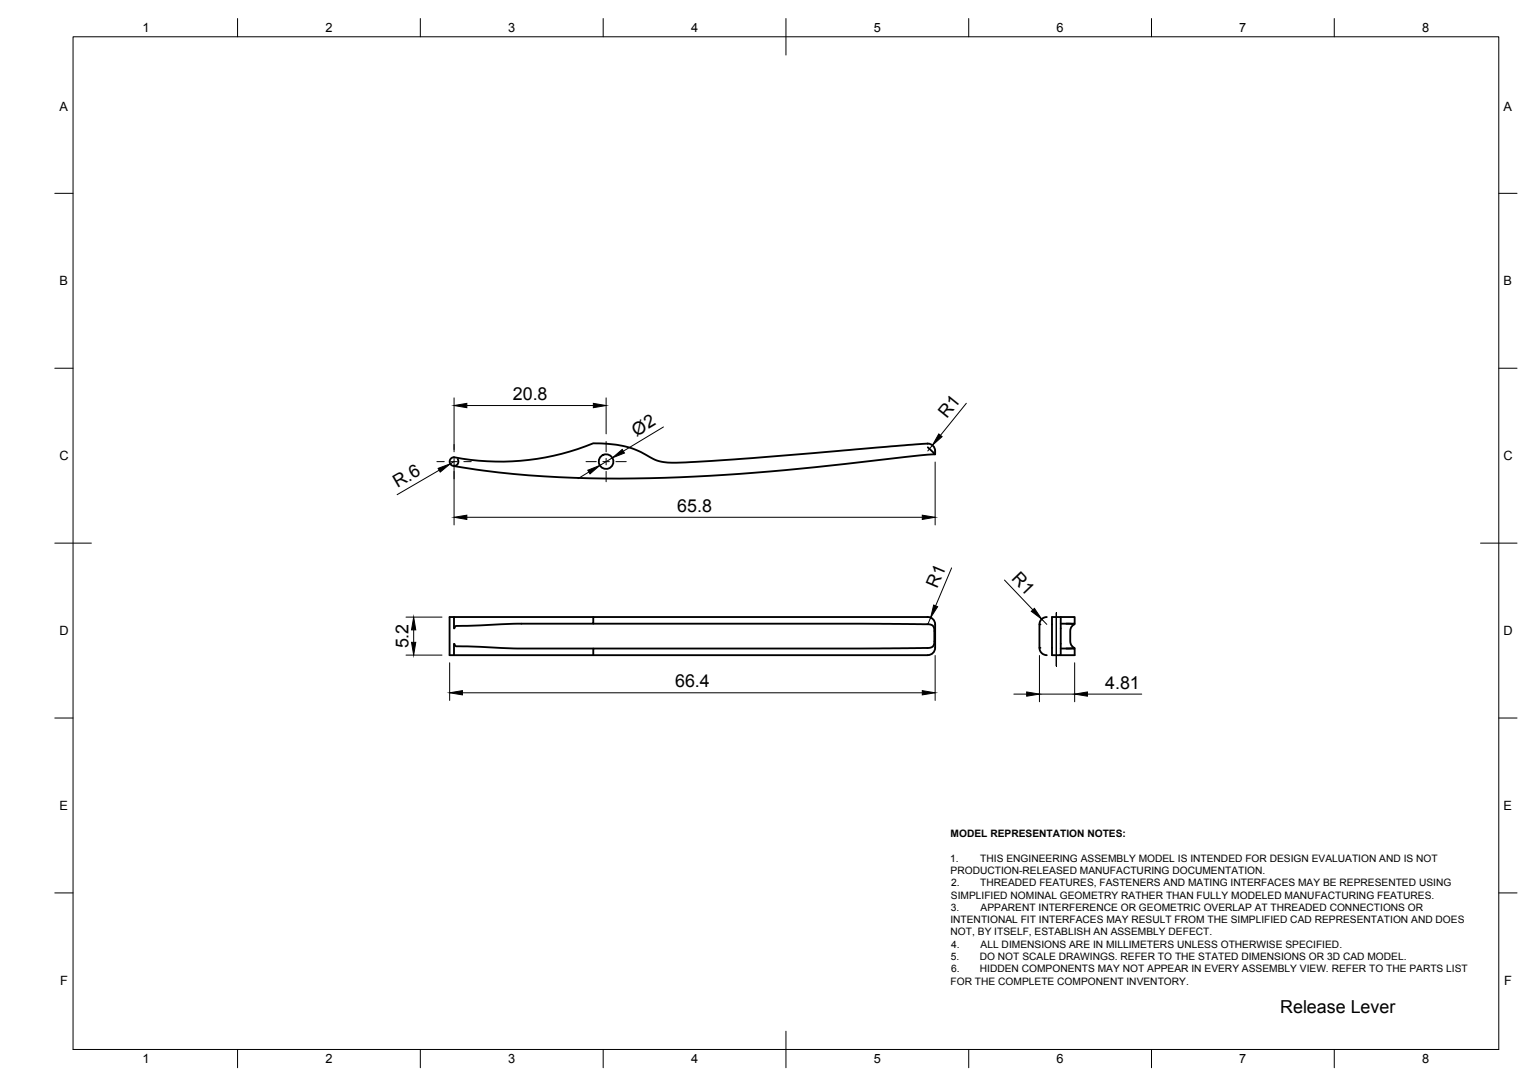
ISO-10303-21;
HEADER;
/* Generated by software containing ST-Developer
 * from STEP Tools, Inc. (www.steptools.com) 
 */

FILE_DESCRIPTION(
/* description */ ('STEP AP214'),
/* implementation_level */ '2;1');

FILE_NAME(
/* name */ 'Release Lever.step',
/* time_stamp */ '2026-10-06T11:11:25-07:00',
/* author */ (''),
/* organization */ (''),
/* preprocessor_version */ 'ST-DEVELOPER v20.2',
/* originating_system */ 'Autodesk Translation Framework v15.15.0.0',
/* authorisation */ '');

FILE_SCHEMA (('AUTOMOTIVE_DESIGN { 1 0 10303 214 3 1 1 }'));
ENDSEC;

DATA;
#10=MECHANICAL_DESIGN_GEOMETRIC_PRESENTATION_REPRESENTATION('',(#708),#47717);
#121=ELLIPSE('',#9861,992.32273705942,143.940737429079);
#122=ELLIPSE('',#9863,1.41421356237156,0.999999999998736);
#123=ELLIPSE('',#9865,1.41421356237466,1.00000000000111);
#133=B_SPLINE_SURFACE_WITH_KNOTS('',3,1,((#46101,#46102),(#46103,#46104),
(#46105,#46106),(#46107,#46108),(#46109,#46110),(#46111,#46112)),
 .UNSPECIFIED.,.F.,.F.,.F.,(4,1,1,4),(2,2),(0.0598879849550618,0.738151675687099,
0.838151675687099,1.),(0.,0.118332698778717),.UNSPECIFIED.);
#134=B_SPLINE_SURFACE_WITH_KNOTS('',3,1,((#46331,#46332),(#46333,#46334),
(#46335,#46336),(#46337,#46338)),.UNSPECIFIED.,.F.,.F.,.F.,(4,4),(2,2),
(0.,0.99999999993505),(0.,0.384000000000005),.UNSPECIFIED.);
#135=B_SPLINE_SURFACE_WITH_KNOTS('',3,1,((#46385,#46386),(#46387,#46388),
(#46389,#46390),(#46391,#46392),(#46393,#46394),(#46395,#46396)),
 .UNSPECIFIED.,.F.,.F.,.F.,(4,1,1,4),(2,2),(0.0598879849550605,0.738151675687099,
0.838151675687099,1.),(0.,0.118332698778627),.UNSPECIFIED.);
#136=B_SPLINE_SURFACE_WITH_KNOTS('',3,1,((#46513,#46514),(#46515,#46516),
(#46517,#46518),(#46519,#46520),(#46521,#46522),(#46523,#46524),(#46525,
#46526),(#46527,#46528),(#46529,#46530),(#46531,#46532),(#46533,#46534),
(#46535,#46536),(#46537,#46538),(#46539,#46540),(#46541,#46542),(#46543,
#46544),(#46545,#46546),(#46547,#46548),(#46549,#46550),(#46551,#46552),
(#46553,#46554),(#46555,#46556)),.UNSPECIFIED.,.F.,.F.,.F.,(4,2,1,1,2,2,
2,2,2,2,2,4),(2,2),(0.,0.00781250000000001,0.015625,0.03125,0.0624999999999999,
0.125,0.25,0.5,0.749999999999999,0.874999999999999,0.9375,1.),(0.,0.412896000000006),
 .UNSPECIFIED.);
#489=B_SPLINE_CURVE_WITH_KNOTS('',3,(#45956,#45957,#45958,#45959,#45960,
#45961),.UNSPECIFIED.,.F.,.F.,(4,2,4),(9.99994026930247E-7,0.0176151554172842,
0.0352487921890912),.UNSPECIFIED.);
#490=B_SPLINE_CURVE_WITH_KNOTS('',3,(#45963,#45964,#45965,#45966,#45967,
#45968,#45969,#45970,#45971,#45972,#45973,#45974,#45975,#45976,#45977,#45978,
#45979,#45980,#45981,#45982,#45983,#45984,#45985,#45986,#45987,#45988,#45989,
#45990,#45991,#45992,#45993,#45994,#45995,#45996,#45997,#45998,#45999,#46000,
#46001,#46002,#46003,#46004,#46005,#46006,#46007,#46008,#46009,#46010,#46011,
#46012,#46013,#46014),.UNSPECIFIED.,.F.,.F.,(4,3,3,3,3,3,3,3,3,3,3,3,3,
3,3,3,3,4),(0.000349648495401886,0.000435856450628066,0.000518346998497937,
0.000600826327770219,0.000683750987549706,0.000694480316306607,0.000804774657733104,
0.000922043397533562,0.00103931213733402,0.00116300366655803,0.00129638856133148,
0.00138414395836143,0.00145781361132506,0.0015307723859531,0.00155655986887515,
0.00162456036766277,0.00169016314809249,0.00172897577938886),
 .UNSPECIFIED.);
#491=B_SPLINE_CURVE_WITH_KNOTS('',3,(#46018,#46019,#46020,#46021,#46022,
#46023,#46024,#46025,#46026,#46027,#46028,#46029,#46030,#46031,#46032,#46033,
#46034,#46035,#46036,#46037,#46038,#46039,#46040,#46041,#46042,#46043,#46044,
#46045,#46046,#46047,#46048,#46049,#46050,#46051,#46052,#46053,#46054,#46055,
#46056,#46057,#46058,#46059,#46060,#46061,#46062,#46063,#46064,#46065,#46066,
#46067,#46068,#46069,#46070,#46071,#46072,#46073,#46074,#46075),
 .UNSPECIFIED.,.F.,.F.,(4,3,3,3,3,3,3,3,3,3,3,3,3,3,3,3,3,3,3,4),(0.,6.18208684431606E-5,
0.000125984546932246,0.00017272653853377,0.000254497619285616,0.000336923412298459,
0.00034545307706754,0.000446850586818363,0.000547260798830634,0.000644898132372486,
0.000690906154135026,0.000804288074237915,0.000913238839396781,0.00101713942033291,
0.00103635923120251,0.00112272247834549,0.00120469306612868,0.0012867711835707,
0.00136943274587814,0.00138181221977441),.UNSPECIFIED.);
#492=B_SPLINE_CURVE_WITH_KNOTS('',3,(#46076,#46077,#46078,#46079,#46080,
#46081),.UNSPECIFIED.,.F.,.F.,(4,2,4),(2.506792132088E-5,0.0175792343156468,
0.0353218856598025),.UNSPECIFIED.);
#493=B_SPLINE_CURVE_WITH_KNOTS('',3,(#46115,#46116,#46117,#46118,#46119,
#46120),.UNSPECIFIED.,.F.,.F.,(4,1,1,4),(0.376076502031257,0.738151675687099,
0.838151675687099,1.),.UNSPECIFIED.);
#494=B_SPLINE_CURVE_WITH_KNOTS('',3,(#46122,#46123,#46124,#46125,#46126,
#46127),.UNSPECIFIED.,.F.,.F.,(4,2,4),(-0.64239307361528,-0.386347437361555,
-6.40648423200219E-10),.UNSPECIFIED.);
#495=B_SPLINE_CURVE_WITH_KNOTS('',3,(#46131,#46132,#46133,#46134,#46135,
#46136),.UNSPECIFIED.,.F.,.F.,(4,1,1,4),(0.0598879851737023,0.738151675687099,
0.838151675687099,1.),.UNSPECIFIED.);
#496=B_SPLINE_CURVE_WITH_KNOTS('',3,(#46142,#46143,#46144,#46145,#46146,
#46147,#46148,#46149,#46150,#46151,#46152,#46153),.UNSPECIFIED.,.F.,.F.,
(4,2,2,2,2,4),(-0.843680482904519,-0.817052168712459,-0.771952825368238,
-0.653804262290151,-0.443525213357367,-1.91323158427181E-7),
 .UNSPECIFIED.);
#497=B_SPLINE_CURVE_WITH_KNOTS('',3,(#46161,#46162,#46163,#46164,#46165,
#46166),.UNSPECIFIED.,.F.,.F.,(4,1,1,4),(0.0598879851737348,0.738151675687099,
0.838151675687099,1.),.UNSPECIFIED.);
#498=B_SPLINE_CURVE_WITH_KNOTS('',3,(#46168,#46169,#46170,#46171,#46172,
#46173,#46174,#46175,#46176,#46177,#46178,#46179,#46180,#46181,#46182,#46183,
#46184,#46185,#46186,#46187,#46188,#46189,#46190,#46191,#46192,#46193,#46194,
#46195,#46196,#46197,#46198,#46199,#46200,#46201,#46202,#46203,#46204,#46205,
#46206,#46207,#46208,#46209,#46210,#46211,#46212,#46213,#46214,#46215,#46216,
#46217,#46218,#46219,#46220,#46221,#46222,#46223,#46224,#46225,#46226,#46227,
#46228,#46229,#46230,#46231,#46232,#46233,#46234,#46235,#46236,#46237,#46238,
#46239,#46240,#46241,#46242,#46243,#46244,#46245,#46246),.UNSPECIFIED.,
 .F.,.F.,(4,3,3,3,3,3,3,3,3,3,3,3,3,3,3,3,3,3,3,3,3,3,3,3,3,3,4),(0.,0.00133019741218274,
0.00338235256079639,0.00652827854954051,0.00749519144790343,0.00804058416816147,
0.0120370484455271,0.0157490242005424,0.0160811683363229,0.0208199774885995,
0.024033074620882,0.0241217525044844,0.0295749122668503,0.0321623366726459,
0.0323411021984972,0.0384974117946658,0.0449050664554913,0.0482435050089688,
0.0490120029708162,0.0550890503579654,0.0562840891771302,0.0573667064243252,
0.060304381261211,0.0615453779150555,0.0623145273032513,0.063632912088931,
0.0643246733452917),.UNSPECIFIED.);
#499=B_SPLINE_CURVE_WITH_KNOTS('',3,(#46252,#46253,#46254,#46255,#46256,
#46257,#46258,#46259,#46260,#46261,#46262,#46263,#46264,#46265,#46266,#46267,
#46268,#46269,#46270,#46271,#46272,#46273,#46274,#46275,#46276,#46277,#46278,
#46279,#46280,#46281,#46282,#46283,#46284,#46285,#46286,#46287,#46288,#46289,
#46290,#46291,#46292,#46293,#46294,#46295,#46296,#46297,#46298,#46299,#46300,
#46301,#46302,#46303,#46304,#46305,#46306,#46307,#46308,#46309,#46310,#46311,
#46312,#46313,#46314,#46315,#46316,#46317,#46318,#46319,#46320,#46321,#46322,
#46323,#46324,#46325,#46326,#46327,#46328,#46329,#46330),.UNSPECIFIED.,
 .F.,.F.,(4,3,3,3,3,3,3,3,3,3,3,3,3,3,3,3,3,3,3,3,3,3,3,3,3,3,4),(0.,0.000694963224053612,
0.00201945044095915,0.00279216000467784,0.0040389008819183,0.0069901733868374,
0.00807780176383661,0.0141829780064518,0.0153835484055692,0.0161556035276732,
0.0226284612866144,0.0288382348705923,0.0321316140743103,0.0323112070553464,
0.0377896082937388,0.040389008819183,0.0404780971676904,0.0452388410930198,
0.0484668105830197,0.0488004921202978,0.0528154549227909,0.0565446123468563,
0.0570925295361479,0.0602530171328019,0.0612244055941231,0.063286059589963,
0.0646224141106929),.UNSPECIFIED.);
#500=B_SPLINE_CURVE_WITH_KNOTS('',3,(#46339,#46340,#46341,#46342,#46343,
#46344,#46345,#46346,#46347,#46348,#46349,#46350,#46351,#46352,#46353,#46354,
#46355,#46356,#46357,#46358,#46359,#46360),.UNSPECIFIED.,.F.,.F.,(4,2,2,
2,2,2,2,2,2,2,4),(0.,0.00822683057377827,0.0164536611475565,0.0246804917213348,
0.0329073222951131,0.0493609834426696,0.0575878140164479,0.061701229303337,
0.0637579369467816,0.0647862907685039,0.0658146445902262),.UNSPECIFIED.);
#501=B_SPLINE_CURVE_WITH_KNOTS('',3,(#46361,#46362,#46363,#46364,#46365,
#46366,#46367,#46368,#46369,#46370,#46371,#46372,#46373,#46374,#46375,#46376,
#46377,#46378,#46379,#46380,#46381,#46382,#46383,#46384),.UNSPECIFIED.,
 .F.,.F.,(4,2,2,2,2,2,2,2,2,2,2,4),(-6.00000000093941E-8,0.00051597907764729,
0.00103201815529459,0.00206409631058923,0.00412825262117847,0.0082565652423569,
0.0165131904847138,0.0330264409694275,0.0412830662117844,0.0495396914541413,
0.0577963166964982,0.0660529419388551),.UNSPECIFIED.);
#502=B_SPLINE_CURVE_WITH_KNOTS('',3,(#46400,#46401,#46402,#46403,#46404,
#46405),.UNSPECIFIED.,.F.,.F.,(4,2,4),(-1.76748570019267,-0.704486820958434,
-1.00000183531384E-6),.UNSPECIFIED.);
#503=B_SPLINE_CURVE_WITH_KNOTS('',3,(#46407,#46408,#46409,#46410,#46411,
#46412),.UNSPECIFIED.,.F.,.F.,(4,1,1,4),(0.376076502030214,0.738151675687099,
0.838151675687099,1.),.UNSPECIFIED.);
#504=B_SPLINE_CURVE_WITH_KNOTS('',3,(#46417,#46418,#46419,#46420,#46421,
#46422,#46423,#46424,#46425,#46426,#46427,#46428),.UNSPECIFIED.,.F.,.F.,
(4,2,2,2,2,4),(-0.957807021571877,-0.464707050841796,-0.230924084318286,
-0.0995694788423429,-0.0494291617315582,-0.0198244706793161),
 .UNSPECIFIED.);
#505=B_SPLINE_CURVE_WITH_KNOTS('',3,(#46430,#46431,#46432,#46433,#46434,
#46435,#46436,#46437,#46438,#46439,#46440,#46441,#46442,#46443,#46444,#46445,
#46446,#46447,#46448,#46449,#46450,#46451,#46452,#46453,#46454,#46455,#46456,
#46457),.UNSPECIFIED.,.F.,.F.,(4,3,3,3,3,3,3,3,3,4),(2.77555756156289E-17,
0.00571779521669806,0.00742042674236585,0.00752642944116232,0.0140544642997195,
0.0148408534847317,0.0186294855440519,0.0236729311553377,0.0285768772393396,
0.0296817069694633),.UNSPECIFIED.);
#506=B_SPLINE_CURVE_WITH_KNOTS('',3,(#46458,#46459,#46460,#46461,#46462,
#46463,#46464,#46465,#46466,#46467,#46468,#46469,#46470),.UNSPECIFIED.,
 .F.,.F.,(4,3,3,3,4),(0.0315167029732621,0.0353810056968997,0.0390981239403465,
0.0415114270041217,0.0422033631272556),.UNSPECIFIED.);
#507=B_SPLINE_CURVE_WITH_KNOTS('',3,(#46472,#46473,#46474,#46475,#46476,
#46477,#46478,#46479,#46480,#46481,#46482,#46483,#46484),.UNSPECIFIED.,
 .F.,.F.,(4,3,3,3,4),(0.,0.000690309032879575,0.00438171613044424,0.00821369103151036,
0.0106615304346148),.UNSPECIFIED.);
#508=B_SPLINE_CURVE_WITH_KNOTS('',3,(#46485,#46486,#46487,#46488,#46489,
#46490,#46491,#46492,#46493,#46494,#46495,#46496,#46497,#46498,#46499,#46500,
#46501,#46502,#46503,#46504,#46505,#46506,#46507,#46508,#46509,#46510,#46511,
#46512),.UNSPECIFIED.,.F.,.F.,(4,3,3,3,3,3,3,3,3,4),(0.0124922114387784,
0.0173786759880834,0.0224014774550337,0.0235184435261858,0.0272981666037043,
0.0338108507614971,0.0345953907531371,0.0347011441861673,0.0404054939590322,
0.0421041217686302),.UNSPECIFIED.);
#509=B_SPLINE_CURVE_WITH_KNOTS('',3,(#46558,#46559,#46560,#46561,#46562,
#46563,#46564,#46565,#46566,#46567,#46568,#46569),.UNSPECIFIED.,.F.,.F.,
(4,2,1,1,2,2,4),(0.,0.00781250000000001,0.015625,0.03125,0.0624999999999999,
0.125,0.242820560992689),.UNSPECIFIED.);
#510=B_SPLINE_CURVE_WITH_KNOTS('',3,(#46571,#46572,#46573,#46574,#46575,
#46576,#46577,#46578,#46579,#46580,#46581,#46582,#46583,#46584,#46585,#46586,
#46587,#46588,#46589,#46590,#46591,#46592,#46593,#46594,#46595,#46596,#46597,
#46598,#46599,#46600,#46601,#46602,#46603,#46604,#46605,#46606,#46607,#46608,
#46609,#46610,#46611,#46612,#46613,#46614,#46615,#46616,#46617,#46618,#46619,
#46620,#46621,#46622,#46623,#46624,#46625,#46626,#46627,#46628),
 .UNSPECIFIED.,.F.,.F.,(4,3,3,3,3,3,3,3,3,3,3,3,3,3,3,3,3,3,3,4),(0.,0.000180857725498468,
0.000242475536420596,0.000462636248961816,0.000484380312649641,0.000484543019812994,
0.000726570468974455,0.000726736566375218,0.000847847927148936,0.000968760625299268,
0.000968976684750301,0.00109011139518026,0.00121095078162408,0.00121122083086588,
0.00145314093794889,0.00145337525175495,0.00167755435588957,0.00169564548526077,
0.00188459038844521,0.00193752125059852),.UNSPECIFIED.);
#511=B_SPLINE_CURVE_WITH_KNOTS('',3,(#46630,#46631,#46632,#46633,#46634,
#46635,#46636,#46637,#46638,#46639,#46640,#46641,#46642,#46643,#46644,#46645,
#46646,#46647),.UNSPECIFIED.,.F.,.F.,(4,2,2,2,2,2,2,2,4),(0.0216871878151901,
0.032680217438002,0.0436732470608138,0.0546662766836257,0.0601627914950316,
0.0629110489007346,0.0642851776035861,0.0649722419550118,0.0656593063064375),
 .UNSPECIFIED.);
#512=B_SPLINE_CURVE_WITH_KNOTS('',3,(#46651,#46652,#46653,#46654,#46655,
#46656,#46657,#46658,#46659,#46660,#46661,#46662,#46663,#46664,#46665,#46666,
#46667,#46668),.UNSPECIFIED.,.F.,.F.,(4,2,2,2,2,2,2,2,4),(0.,0.000689842611306874,
0.00137968522261375,0.00275937044522753,0.00551874089045509,0.0110374817809102,
0.0220749635618205,0.0331124453427309,0.0441499271236412),.UNSPECIFIED.);
#513=B_SPLINE_CURVE_WITH_KNOTS('',3,(#46670,#46671,#46672,#46673,#46674,
#46675,#46676,#46677,#46678,#46679,#46680,#46681,#46682,#46683,#46684,#46685,
#46686,#46687,#46688,#46689,#46690,#46691,#46692,#46693,#46694,#46695,#46696,
#46697,#46698,#46699,#46700,#46701,#46702,#46703,#46704,#46705,#46706,#46707,
#46708,#46709,#46710,#46711,#46712,#46713,#46714,#46715,#46716,#46717,#46718,
#46719,#46720,#46721,#46722,#46723,#46724),.UNSPECIFIED.,.F.,.F.,(4,3,3,
3,3,3,3,3,3,3,3,3,3,3,3,3,3,3,4),(9.33050753687133E-16,0.00018425279266257,
0.000235878931742768,0.000454457410544906,0.000472142579138733,0.000472396351922799,
0.000708293271574268,0.000708594527884195,0.000826400049535313,0.000944531464697737,
0.000944792703845591,0.00106266228766045,0.00118075303404218,0.00118099087980699,
0.0014168040003498,0.00141718905576838,0.00165316656365015,0.001850849561933,
0.00188958540769117),.UNSPECIFIED.);
#514=B_SPLINE_CURVE_WITH_KNOTS('',3,(#46828,#46829,#46830,#46831,#46832,
#46833,#46834,#46835,#46836,#46837,#46838,#46839,#46840,#46841,#46842,#46843,
#46844,#46845,#46846,#46847,#46848,#46849,#46850,#46851,#46852,#46853,#46854,
#46855,#46856,#46857,#46858,#46859,#46860,#46861,#46862,#46863,#46864,#46865,
#46866,#46867,#46868,#46869,#46870,#46871,#46872,#46873,#46874,#46875,#46876),
 .UNSPECIFIED.,.F.,.F.,(4,3,3,3,3,3,3,3,3,3,3,3,3,3,3,3,4),(0.,0.000109468558295443,
0.000219785271344123,0.000330646009385498,0.00044249674566146,0.000468452330512348,
0.000589929933612792,0.000715263674224842,0.000847107675387793,0.000936904661024695,
0.00105512166097558,0.0011758327883036,0.00129946242311971,0.00140535699153704,
0.00158825025111182,0.00178591157987006,0.00187380932204939),
 .UNSPECIFIED.);
#515=B_SPLINE_CURVE_WITH_KNOTS('',3,(#46979,#46980,#46981,#46982,#46983,
#46984,#46985,#46986,#46987,#46988,#46989,#46990,#46991,#46992,#46993,#46994,
#46995,#46996,#46997,#46998,#46999,#47000,#47001,#47002,#47003,#47004,#47005,
#47006,#47007,#47008,#47009,#47010,#47011,#47012,#47013,#47014,#47015,#47016,
#47017,#47018,#47019,#47020,#47021,#47022,#47023,#47024,#47025,#47026,#47027),
 .UNSPECIFIED.,.F.,.F.,(4,3,3,3,3,3,3,3,3,3,3,3,3,3,3,3,4),(-6.33283738354695E-6,
0.000175132894873384,0.000348429481852089,0.000462988112447956,0.00058681834786203,
0.000709001656163456,0.000827259972155947,0.00093230906227946,0.0010641247249674,
0.00119160914162567,0.00131279282513799,0.00140163001211096,0.00151896024956884,
0.0016299235561327,0.00174028554103239,0.00184999846319747,0.00187095096194247),
 .UNSPECIFIED.);
#516=B_SPLINE_CURVE_WITH_KNOTS('',3,(#47033,#47034,#47035,#47036,#47037,
#47038,#47039,#47040,#47041,#47042,#47043,#47044,#47045,#47046,#47047,#47048,
#47049,#47050,#47051,#47052),.UNSPECIFIED.,.F.,.F.,(4,2,2,2,2,2,2,2,2,4),
(1.63264169611634E-6,0.00112071490622925,0.00249410485118844,0.00667587597325017,
0.0315279582548989,0.0586878942058162,0.0843353212386066,0.111794096810849,
0.141395316871198,0.169000061137383),.UNSPECIFIED.);
#517=B_SPLINE_CURVE_WITH_KNOTS('',3,(#47053,#47054,#47055,#47056,#47057,
#47058,#47059,#47060,#47061,#47062,#47063,#47064,#47065,#47066,#47067,#47068,
#47069,#47070,#47071,#47072),.UNSPECIFIED.,.F.,.F.,(4,2,2,2,2,2,2,2,2,4),
(0.,0.0273497535277419,0.0569920982606061,0.0844751673709711,0.110215240941746,
0.137351156959471,0.162388202840594,0.166588867976713,0.167966825157961,
0.169089008366351),.UNSPECIFIED.);
#598=(
BOUNDED_SURFACE()
B_SPLINE_SURFACE(3,2,((#46726,#46727,#46728),(#46729,#46730,#46731),(#46732,
#46733,#46734),(#46735,#46736,#46737),(#46738,#46739,#46740),(#46741,#46742,
#46743),(#46744,#46745,#46746),(#46747,#46748,#46749),(#46750,#46751,#46752),
(#46753,#46754,#46755),(#46756,#46757,#46758),(#46759,#46760,#46761),(#46762,
#46763,#46764),(#46765,#46766,#46767),(#46768,#46769,#46770),(#46771,#46772,
#46773),(#46774,#46775,#46776),(#46777,#46778,#46779),(#46780,#46781,#46782),
(#46783,#46784,#46785),(#46786,#46787,#46788),(#46789,#46790,#46791),(#46792,
#46793,#46794),(#46795,#46796,#46797),(#46798,#46799,#46800),(#46801,#46802,
#46803),(#46804,#46805,#46806),(#46807,#46808,#46809),(#46810,#46811,#46812),
(#46813,#46814,#46815),(#46816,#46817,#46818),(#46819,#46820,#46821),(#46822,
#46823,#46824),(#46825,#46826,#46827)),.UNSPECIFIED.,.F.,.F.,.F.)
B_SPLINE_SURFACE_WITH_KNOTS((4,2,2,2,2,2,2,2,2,2,2,2,2,2,2,2,4),(3,3),(0.0462087893288186,
0.0464703270720222,0.0466010959436241,0.046666480379425,0.0467318648152259,
0.0472549403016333,0.048301091274448,0.0503933932200775,0.0545779971113364,
0.0629472048938543,0.07968562045889,0.0880548282414078,0.0964240360239257,
0.104793243806444,0.108977847697702,0.111070149643332,0.113162451588961),
(0.,1.),.UNSPECIFIED.)
GEOMETRIC_REPRESENTATION_ITEM()
RATIONAL_B_SPLINE_SURFACE(((1.,0.707106781186557,1.),(1.,0.707106781186557,
1.),(1.,0.707106781186551,1.),(1.,0.707106781186551,1.),(1.,0.707106781186557,
1.),(1.,0.707106781186557,1.),(1.,0.707106781186557,1.),(1.,0.707106781186557,
1.),(1.,0.707106781186557,1.),(1.,0.707106781186557,1.),(1.,0.707106781186557,
1.),(1.,0.707106781186557,1.),(1.,0.707106781186557,1.),(1.,0.707106781186557,
1.),(1.,0.707106781186562,1.),(1.,0.707106781186562,1.),(1.,0.707106781186557,
1.),(1.,0.707106781186557,1.),(1.,0.707106781186557,1.),(1.,0.707106781186557,
1.),(1.,0.707106781186557,1.),(1.,0.707106781186557,1.),(1.,0.707106781186538,
1.),(1.,0.707106781186538,1.),(1.,0.707106781186557,1.),(1.,0.707106781186557,
1.),(1.,0.707106781186557,1.),(1.,0.707106781186557,1.),(1.,0.707106781186556,
1.),(1.,0.707106781186556,1.),(1.,0.707106781186557,1.),(1.,0.707106781186557,
1.),(1.,0.707106781186548,1.),(1.,0.707106781186548,1.)))
REPRESENTATION_ITEM('')
SURFACE()
);
#599=(
BOUNDED_SURFACE()
B_SPLINE_SURFACE(3,2,((#46877,#46878,#46879),(#46880,#46881,#46882),(#46883,
#46884,#46885),(#46886,#46887,#46888),(#46889,#46890,#46891),(#46892,#46893,
#46894),(#46895,#46896,#46897),(#46898,#46899,#46900),(#46901,#46902,#46903),
(#46904,#46905,#46906),(#46907,#46908,#46909),(#46910,#46911,#46912),(#46913,
#46914,#46915),(#46916,#46917,#46918),(#46919,#46920,#46921),(#46922,#46923,
#46924),(#46925,#46926,#46927),(#46928,#46929,#46930),(#46931,#46932,#46933),
(#46934,#46935,#46936),(#46937,#46938,#46939),(#46940,#46941,#46942),(#46943,
#46944,#46945),(#46946,#46947,#46948),(#46949,#46950,#46951),(#46952,#46953,
#46954),(#46955,#46956,#46957),(#46958,#46959,#46960),(#46961,#46962,#46963),
(#46964,#46965,#46966),(#46967,#46968,#46969),(#46970,#46971,#46972),(#46973,
#46974,#46975),(#46976,#46977,#46978)),.UNSPECIFIED.,.F.,.F.,.F.)
B_SPLINE_SURFACE_WITH_KNOTS((4,2,2,2,2,2,2,2,2,2,2,2,2,2,2,2,4),(3,3),(0.0317072603307532,
0.0337720562518688,0.0358368521729843,0.0399664440152153,0.0482256276996774,
0.0564848113841394,0.0647439950686015,0.0812623624375256,0.0895215461219877,
0.0936511379642187,0.0957159338853342,0.096748331845892,0.0972645308261708,
0.0973290556987057,0.0973935805712406,0.0975226303163103,0.0977807298064497),
(0.,1.),.UNSPECIFIED.)
GEOMETRIC_REPRESENTATION_ITEM()
RATIONAL_B_SPLINE_SURFACE(((1.,0.707106781186557,1.),(1.,0.707106781186557,
1.),(1.,0.707106781186557,1.),(1.,0.707106781186557,1.),(1.,0.707106781186557,
1.),(1.,0.707106781186557,1.),(1.,0.707106781186556,1.),(1.,0.707106781186556,
1.),(1.,0.707106781186557,1.),(1.,0.707106781186557,1.),(1.,0.707106781186557,
1.),(1.,0.707106781186557,1.),(1.,0.707106781186557,1.),(1.,0.707106781186557,
1.),(1.,0.707106781186557,1.),(1.,0.707106781186557,1.),(1.,0.707106781186553,
1.),(1.,0.707106781186553,1.),(1.,0.707106781186557,1.),(1.,0.707106781186557,
1.),(1.,0.707106781186557,1.),(1.,0.707106781186557,1.),(1.,0.707106781186557,
1.),(1.,0.707106781186557,1.),(1.,0.707106781186557,1.),(1.,0.707106781186557,
1.),(1.,0.707106781186557,1.),(1.,0.707106781186557,1.),(1.,0.707106781186557,
1.),(1.,0.707106781186557,1.),(1.,0.707106781186557,1.),(1.,0.707106781186557,
1.),(1.,0.707106781186557,1.),(1.,0.707106781186557,1.)))
REPRESENTATION_ITEM('')
SURFACE()
);
#600=(
BOUNDED_SURFACE()
B_SPLINE_SURFACE(3,2,((#47073,#47074,#47075),(#47076,#47077,#47078),(#47079,
#47080,#47081),(#47082,#47083,#47084),(#47085,#47086,#47087),(#47088,#47089,
#47090),(#47091,#47092,#47093),(#47094,#47095,#47096),(#47097,#47098,#47099),
(#47100,#47101,#47102),(#47103,#47104,#47105),(#47106,#47107,#47108),(#47109,
#47110,#47111),(#47112,#47113,#47114),(#47115,#47116,#47117),(#47118,#47119,
#47120),(#47121,#47122,#47123),(#47124,#47125,#47126),(#47127,#47128,#47129),
(#47130,#47131,#47132),(#47133,#47134,#47135),(#47136,#47137,#47138)),
 .UNSPECIFIED.,.F.,.F.,.F.)
B_SPLINE_SURFACE_WITH_KNOTS((4,2,2,2,2,2,2,2,2,2,4),(3,3),(0.0497700329860562,
0.0499435417983895,0.0501170506107227,0.0504640682353892,0.0511581034847222,
0.0525461739833882,0.0553223149807202,0.0608745969753841,0.0719791609647121,
0.08308372495404,0.0941882889433679),(0.,1.),.UNSPECIFIED.)
GEOMETRIC_REPRESENTATION_ITEM()
RATIONAL_B_SPLINE_SURFACE(((1.,0.707106781186552,1.),(1.,0.707106781186552,
1.),(1.,0.707106781186548,1.),(1.,0.707106781186548,1.),(1.,0.707106781186548,
1.),(1.,0.707106781186548,1.),(1.,0.707106781186548,1.),(1.,0.707106781186548,
1.),(1.,0.707106781186548,1.),(1.,0.707106781186548,1.),(1.,0.707106781186552,
1.),(1.,0.707106781186552,1.),(1.,0.707106781186552,1.),(1.,0.707106781186552,
1.),(1.,0.707106781186543,1.),(1.,0.707106781186543,1.),(1.,0.707106781186548,
1.),(1.,0.707106781186548,1.),(1.,0.707106781186548,1.),(1.,0.707106781186548,
1.),(1.,0.707106781186548,1.),(1.,0.707106781186548,1.)))
REPRESENTATION_ITEM('')
SURFACE()
);
#601=(
BOUNDED_SURFACE()
B_SPLINE_SURFACE(3,2,((#47140,#47141,#47142),(#47143,#47144,#47145),(#47146,
#47147,#47148),(#47149,#47150,#47151),(#47152,#47153,#47154),(#47155,#47156,
#47157),(#47158,#47159,#47160),(#47161,#47162,#47163),(#47164,#47165,#47166),
(#47167,#47168,#47169),(#47170,#47171,#47172),(#47173,#47174,#47175),(#47176,
#47177,#47178),(#47179,#47180,#47181),(#47182,#47183,#47184),(#47185,#47186,
#47187),(#47188,#47189,#47190),(#47191,#47192,#47193),(#47194,#47195,#47196),
(#47197,#47198,#47199),(#47200,#47201,#47202),(#47203,#47204,#47205)),
 .UNSPECIFIED.,.F.,.F.,.F.)
B_SPLINE_SURFACE_WITH_KNOTS((4,2,2,2,2,2,2,2,2,2,4),(3,3),(0.00146045554386956,
0.00183455394335381,0.0020667680883163,0.00229898223327879,0.00241508930576004,
0.00253119637824129,0.00264730345072254,0.00276341052320378,0.00299562466816628,
0.00322783881312877,0.00360193721261649),(-0.000683445866355827,1.),
 .UNSPECIFIED.)
GEOMETRIC_REPRESENTATION_ITEM()
RATIONAL_B_SPLINE_SURFACE(((1.00042379451114,0.689957513824106,1.),(1.00040554234364,
0.703310559329287,1.),(1.00038207055231,0.720482212916271,1.),(1.00033118410993,
0.75771006437072,1.),(1.00030837452904,0.77439725351972,1.),(1.00025611113095,
0.812632467645312,1.),(1.00022596681978,0.834685648929338,1.),(1.0001846081175,
0.864943131131046,1.),(1.00017167736853,0.874403096882682,1.),(1.00015246067487,
0.88846177701933,1.),(1.00014653964815,0.892793522236095,1.),(1.00014594005926,
0.89323217357368,1.),(1.0001511099939,0.889449917438278,1.),(1.00016917206089,
0.876235946970749,1.),(1.00018188807499,0.866933078428389,1.),(1.0002231052286,
0.836779151366944,1.),(1.00025373494149,0.814370856578693,1.),(1.00030668059841,
0.775636510873654,1.),(1.00032978588761,0.758732985413562,1.),(1.00038153719649,
0.720872409012061,1.),(1.00040541002051,0.7034073651832,1.),(1.00042487779778,
0.689164995581676,1.)))
REPRESENTATION_ITEM('')
SURFACE()
);
#602=(
BOUNDED_SURFACE()
B_SPLINE_SURFACE(3,2,((#47207,#47208,#47209),(#47210,#47211,#47212),(#47213,
#47214,#47215),(#47216,#47217,#47218),(#47219,#47220,#47221),(#47222,#47223,
#47224),(#47225,#47226,#47227),(#47228,#47229,#47230),(#47231,#47232,#47233),
(#47234,#47235,#47236),(#47237,#47238,#47239),(#47240,#47241,#47242)),
 .UNSPECIFIED.,.F.,.F.,.F.)
B_SPLINE_SURFACE_WITH_KNOTS((4,2,2,2,2,4),(3,3),(0.0960380936069649,0.106151670712726,
0.111208459265607,0.113736853542047,0.115001050680268,0.116265247818488),
(0.,1.),.UNSPECIFIED.)
GEOMETRIC_REPRESENTATION_ITEM()
RATIONAL_B_SPLINE_SURFACE(((1.,0.707106781186548,1.),(1.,0.707106781186548,
1.),(1.,0.707106781186548,1.),(1.,0.707106781186548,1.),(1.,0.707106781186557,
1.),(1.,0.707106781186557,1.),(1.,0.707106781186549,1.),(1.,0.707106781186549,
1.),(1.,0.707106781186548,1.),(1.,0.707106781186548,1.),(1.,0.707106781186548,
1.),(1.,0.707106781186548,1.)))
REPRESENTATION_ITEM('')
SURFACE()
);
#603=(
BOUNDED_SURFACE()
B_SPLINE_SURFACE(3,2,((#47243,#47244,#47245),(#47246,#47247,#47248),(#47249,
#47250,#47251),(#47252,#47253,#47254),(#47255,#47256,#47257),(#47258,#47259,
#47260),(#47261,#47262,#47263),(#47264,#47265,#47266),(#47267,#47268,#47269),
(#47270,#47271,#47272),(#47273,#47274,#47275),(#47276,#47277,#47278),(#47279,
#47280,#47281),(#47282,#47283,#47284),(#47285,#47286,#47287),(#47288,#47289,
#47290),(#47291,#47292,#47293),(#47294,#47295,#47296),(#47297,#47298,#47299),
(#47300,#47301,#47302),(#47303,#47304,#47305),(#47306,#47307,#47308)),
 .UNSPECIFIED.,.F.,.F.,.F.)
B_SPLINE_SURFACE_WITH_KNOTS((4,2,2,2,2,2,2,2,2,2,4),(3,3),(0.057360394545972,
0.0683115303997951,0.0792626662536183,0.0902138021074414,0.095689370034353,
0.0984271539978088,0.0997960459795367,0.100480491970401,0.100822714965833,
0.100993826463549,0.101164937961265),(0.,1.),.UNSPECIFIED.)
GEOMETRIC_REPRESENTATION_ITEM()
RATIONAL_B_SPLINE_SURFACE(((1.,0.707106781186537,1.),(1.,0.707106781186537,
1.),(1.,0.707106781186548,1.),(1.,0.707106781186548,1.),(1.,0.707106781186552,
1.),(1.,0.707106781186552,1.),(1.,0.707106781186548,1.),(1.,0.707106781186548,
1.),(1.,0.707106781186548,1.),(1.,0.707106781186548,1.),(1.,0.707106781186549,
1.),(1.,0.707106781186549,1.),(1.,0.707106781186552,1.),(1.,0.707106781186552,
1.),(1.,0.707106781186548,1.),(1.,0.707106781186548,1.),(1.,0.707106781186552,
1.),(1.,0.707106781186552,1.),(1.,0.707106781186548,1.),(1.,0.707106781186548,
1.),(1.,0.707106781186549,1.),(1.,0.707106781186549,1.)))
REPRESENTATION_ITEM('')
SURFACE()
);
#604=(
BOUNDED_SURFACE()
B_SPLINE_SURFACE(3,2,((#47310,#47311,#47312),(#47313,#47314,#47315),(#47316,
#47317,#47318),(#47319,#47320,#47321),(#47322,#47323,#47324),(#47325,#47326,
#47327),(#47328,#47329,#47330),(#47331,#47332,#47333),(#47334,#47335,#47336),
(#47337,#47338,#47339),(#47340,#47341,#47342),(#47343,#47344,#47345),(#47346,
#47347,#47348),(#47349,#47350,#47351),(#47352,#47353,#47354),(#47355,#47356,
#47357),(#47358,#47359,#47360),(#47361,#47362,#47363),(#47364,#47365,#47366),
(#47367,#47368,#47369),(#47370,#47371,#47372),(#47373,#47374,#47375)),
 .UNSPECIFIED.,.F.,.F.,.F.)
B_SPLINE_SURFACE_WITH_KNOTS((4,2,2,2,2,2,2,2,2,2,4),(3,3),(0.00144383890556605,
0.00183455394336773,0.0020667680883287,0.00229898223328968,0.00241508930577017,
0.00253119637825066,0.00264730345073115,0.00276341052321164,0.00299562466817261,
0.00322783881313359,0.00361855385093527),(0.,1.00015850089284),
 .UNSPECIFIED.)
GEOMETRIC_REPRESENTATION_ITEM()
RATIONAL_B_SPLINE_SURFACE(((1.,0.688364167948368,1.00009878911524),(1.,
0.70195297713868,1.00009448143846),(1.,0.719609110627684,1.00008888441262),
(1.,0.757837166390466,1.00007676605068),(1.,0.774515601665459,1.00007147895692),
(1.,0.812730758117016,1.00005936468408),(1.,0.834772370599585,1.00005237745356),
(1.,0.865013980137201,1.00004279080934),(1.,0.874468983318253,1.00003979355645),
(1.,0.8885202884607,1.00003533926763),(1.,0.89284976130205,1.000033966817),
(1.,0.893288182527816,1.00003382783669),(1.,0.889507910512134,1.00003502618967),
(1.,0.876300871913868,1.00003921284449),(1.,0.867002883530373,1.00004216032341),
(1.,0.836864774809164,1.00005171415769),(1.,0.814468235110218,1.00005881390077),
(1.,0.775754208917403,1.0000710863162),(1.,0.758859550818501,1.00007644195299),
(1.,0.719981770628353,1.00008876627873),(1.,0.702023873648148,1.00009445896414),
(1.,0.687450036010001,1.0000990788967)))
REPRESENTATION_ITEM('')
SURFACE()
);
#605=(
BOUNDED_SURFACE()
B_SPLINE_SURFACE(3,2,((#47377,#47378,#47379),(#47380,#47381,#47382),(#47383,
#47384,#47385),(#47386,#47387,#47388),(#47389,#47390,#47391),(#47392,#47393,
#47394),(#47395,#47396,#47397),(#47398,#47399,#47400),(#47401,#47402,#47403),
(#47404,#47405,#47406),(#47407,#47408,#47409),(#47410,#47411,#47412)),
 .UNSPECIFIED.,.F.,.F.,.F.)
B_SPLINE_SURFACE_WITH_KNOTS((4,2,2,2,2,4),(3,3),(0.0355884658045091,0.0368351959435732,
0.0380819260826373,0.0405753863607654,0.0455623069170217,0.0555361480295343),
(0.,1.),.UNSPECIFIED.)
GEOMETRIC_REPRESENTATION_ITEM()
RATIONAL_B_SPLINE_SURFACE(((1.,0.707106781186548,1.),(1.,0.707106781186548,
1.),(1.,0.707106781186548,1.),(1.,0.707106781186548,1.),(1.,0.707106781186548,
1.),(1.,0.707106781186548,1.),(1.,0.707106781186567,1.),(1.,0.707106781186567,
1.),(1.,0.707106781186548,1.),(1.,0.707106781186548,1.),(1.,0.707106781186548,
1.),(1.,0.707106781186548,1.)))
REPRESENTATION_ITEM('')
SURFACE()
);
#684=SHAPE_REPRESENTATION_RELATIONSHIP('SRR','None',#47771,#696);
#696=ADVANCED_BREP_SHAPE_REPRESENTATION('',(#720),#47715);
#708=STYLED_ITEM('',(#47830),#720);
#720=MANIFOLD_SOLID_BREP('Body1',#8935);
#753=FACE_BOUND('',#3068,.T.);
#754=FACE_BOUND('',#3070,.T.);
#873=PLANE('',#9848);
#874=PLANE('',#9852);
#875=PLANE('',#9855);
#876=PLANE('',#9859);
#877=PLANE('',#9860);
#1331=LINE('',#45937,#1818);
#1332=LINE('',#45948,#1819);
#1333=LINE('',#45950,#1820);
#1334=LINE('',#45952,#1821);
#1335=LINE('',#46016,#1822);
#1336=LINE('',#46087,#1823);
#1337=LINE('',#46095,#1824);
#1338=LINE('',#46097,#1825);
#1339=LINE('',#46099,#1826);
#1340=LINE('',#46100,#1827);
#1341=LINE('',#46129,#1828);
#1342=LINE('',#46137,#1829);
#1343=LINE('',#46157,#1830);
#1344=LINE('',#46251,#1831);
#1345=LINE('',#46398,#1832);
#1346=LINE('',#46413,#1833);
#1347=LINE('',#46649,#1834);
#1818=VECTOR('',#11938,0.999999999999998);
#1819=VECTOR('',#11949,1000.);
#1820=VECTOR('',#11950,10.);
#1821=VECTOR('',#11951,1000.);
#1822=VECTOR('',#11954,1000.);
#1823=VECTOR('',#11959,0.999999999999998);
#1824=VECTOR('',#11968,1000.);
#1825=VECTOR('',#11969,1000.);
#1826=VECTOR('',#11970,1000.);
#1827=VECTOR('',#11971,1000.);
#1828=VECTOR('',#11972,1000.);
#1829=VECTOR('',#11973,1000.);
#1830=VECTOR('',#11982,1000.);
#1831=VECTOR('',#11991,1000.);
#1832=VECTOR('',#11992,1000.);
#1833=VECTOR('',#11993,1000.);
#1834=VECTOR('',#12002,1000.);
#2042=CYLINDRICAL_SURFACE('',#9835,0.999999999999998);
#2043=CYLINDRICAL_SURFACE('',#9840,0.6);
#2044=CYLINDRICAL_SURFACE('',#9843,0.999999999999998);
#2045=CYLINDRICAL_SURFACE('',#9849,33.6360679582853);
#2046=CYLINDRICAL_SURFACE('',#9857,33.6360679582853);
#2047=CYLINDRICAL_SURFACE('',#9862,1.);
#2048=CYLINDRICAL_SURFACE('',#9864,1.);
#2049=CYLINDRICAL_SURFACE('',#9866,0.999999999999998);
#2518=FACE_OUTER_BOUND('',#3061,.T.);
#2519=FACE_OUTER_BOUND('',#3062,.T.);
#2520=FACE_OUTER_BOUND('',#3063,.T.);
#2521=FACE_OUTER_BOUND('',#3064,.T.);
#2522=FACE_OUTER_BOUND('',#3065,.T.);
#2523=FACE_OUTER_BOUND('',#3066,.T.);
#2524=FACE_OUTER_BOUND('',#3067,.T.);
#2525=FACE_OUTER_BOUND('',#3069,.T.);
#2526=FACE_OUTER_BOUND('',#3071,.T.);
#2527=FACE_OUTER_BOUND('',#3072,.T.);
#2528=FACE_OUTER_BOUND('',#3073,.T.);
#2529=FACE_OUTER_BOUND('',#3074,.T.);
#2530=FACE_OUTER_BOUND('',#3075,.T.);
#2531=FACE_OUTER_BOUND('',#3076,.T.);
#2532=FACE_OUTER_BOUND('',#3077,.T.);
#2533=FACE_OUTER_BOUND('',#3078,.T.);
#2534=FACE_OUTER_BOUND('',#3079,.T.);
#2535=FACE_OUTER_BOUND('',#3080,.T.);
#2536=FACE_OUTER_BOUND('',#3081,.T.);
#2537=FACE_OUTER_BOUND('',#3082,.T.);
#2538=FACE_OUTER_BOUND('',#3083,.T.);
#2539=FACE_OUTER_BOUND('',#3084,.T.);
#2540=FACE_OUTER_BOUND('',#3085,.T.);
#2541=FACE_OUTER_BOUND('',#3086,.T.);
#2542=FACE_OUTER_BOUND('',#3087,.T.);
#3061=EDGE_LOOP('',(#8125,#8126,#8127,#8128,#8129,#8130));
#3062=EDGE_LOOP('',(#8131,#8132,#8133,#8134,#8135,#8136,#8137,#8138,#8139,
#8140));
#3063=EDGE_LOOP('',(#8141,#8142,#8143,#8144,#8145,#8146));
#3064=EDGE_LOOP('',(#8147,#8148,#8149,#8150));
#3065=EDGE_LOOP('',(#8151,#8152,#8153,#8154,#8155));
#3066=EDGE_LOOP('',(#8156,#8157,#8158,#8159,#8160));
#3067=EDGE_LOOP('',(#8161,#8162,#8163,#8164,#8165,#8166));
#3068=EDGE_LOOP('',(#8167));
#3069=EDGE_LOOP('',(#8168,#8169,#8170,#8171,#8172,#8173));
#3070=EDGE_LOOP('',(#8174));
#3071=EDGE_LOOP('',(#8175,#8176,#8177,#8178));
#3072=EDGE_LOOP('',(#8179,#8180,#8181,#8182,#8183));
#3073=EDGE_LOOP('',(#8184,#8185,#8186,#8187,#8188));
#3074=EDGE_LOOP('',(#8189,#8190,#8191,#8192,#8193,#8194));
#3075=EDGE_LOOP('',(#8195,#8196,#8197,#8198,#8199,#8200));
#3076=EDGE_LOOP('',(#8201,#8202,#8203,#8204,#8205,#8206,#8207,#8208));
#3077=EDGE_LOOP('',(#8209,#8210,#8211,#8212,#8213));
#3078=EDGE_LOOP('',(#8214,#8215,#8216,#8217,#8218));
#3079=EDGE_LOOP('',(#8219,#8220,#8221,#8222));
#3080=EDGE_LOOP('',(#8223,#8224,#8225,#8226));
#3081=EDGE_LOOP('',(#8227,#8228,#8229,#8230,#8231,#8232,#8233,#8234,#8235,
#8236));
#3082=EDGE_LOOP('',(#8237,#8238,#8239,#8240,#8241));
#3083=EDGE_LOOP('',(#8242,#8243,#8244,#8245));
#3084=EDGE_LOOP('',(#8246,#8247,#8248,#8249));
#3085=EDGE_LOOP('',(#8250,#8251,#8252,#8253,#8254));
#3086=EDGE_LOOP('',(#8255,#8256,#8257,#8258));
#3087=EDGE_LOOP('',(#8259,#8260,#8261,#8262));
#3472=CIRCLE('',#9836,0.999999999999998);
#3473=CIRCLE('',#9837,1.);
#3474=CIRCLE('',#9838,0.999999999999998);
#3475=CIRCLE('',#9839,1.);
#3476=CIRCLE('',#9841,0.6);
#3477=CIRCLE('',#9842,0.6);
#3478=CIRCLE('',#9844,1.);
#3479=CIRCLE('',#9845,0.999999999999998);
#3480=CIRCLE('',#9846,1.);
#3481=CIRCLE('',#9847,0.999999999999998);
#3482=CIRCLE('',#9850,33.6360679582853);
#3483=CIRCLE('',#9851,33.6360679582853);
#3484=CIRCLE('',#9853,0.999999999999998);
#3485=CIRCLE('',#9854,33.6360679582853);
#3486=CIRCLE('',#9856,0.999999999999998);
#3487=CIRCLE('',#9858,33.6360679582853);
#3488=CIRCLE('',#9867,0.999999999999997);
#3489=CIRCLE('',#9868,0.999999999999999);
#3490=CIRCLE('',#9869,1.);
#3491=CIRCLE('',#9870,1.);
#4305=VERTEX_POINT('',#45934);
#4306=VERTEX_POINT('',#45936);
#4307=VERTEX_POINT('',#45938);
#4308=VERTEX_POINT('',#45940);
#4309=VERTEX_POINT('',#45944);
#4310=VERTEX_POINT('',#45945);
#4311=VERTEX_POINT('',#45947);
#4312=VERTEX_POINT('',#45949);
#4313=VERTEX_POINT('',#45951);
#4314=VERTEX_POINT('',#45953);
#4315=VERTEX_POINT('',#45955);
#4316=VERTEX_POINT('',#45962);
#4317=VERTEX_POINT('',#46015);
#4318=VERTEX_POINT('',#46017);
#4319=VERTEX_POINT('',#46083);
#4320=VERTEX_POINT('',#46084);
#4321=VERTEX_POINT('',#46086);
#4322=VERTEX_POINT('',#46089);
#4323=VERTEX_POINT('',#46093);
#4324=VERTEX_POINT('',#46094);
#4325=VERTEX_POINT('',#46096);
#4326=VERTEX_POINT('',#46098);
#4327=VERTEX_POINT('',#46113);
#4328=VERTEX_POINT('',#46114);
#4329=VERTEX_POINT('',#46121);
#4330=VERTEX_POINT('',#46128);
#4331=VERTEX_POINT('',#46130);
#4332=VERTEX_POINT('',#46139);
#4333=VERTEX_POINT('',#46155);
#4334=VERTEX_POINT('',#46156);
#4335=VERTEX_POINT('',#46158);
#4336=VERTEX_POINT('',#46160);
#4337=VERTEX_POINT('',#46248);
#4338=VERTEX_POINT('',#46250);
#4339=VERTEX_POINT('',#46397);
#4340=VERTEX_POINT('',#46399);
#4341=VERTEX_POINT('',#46406);
#4342=VERTEX_POINT('',#46415);
#4343=VERTEX_POINT('',#46557);
#4344=VERTEX_POINT('',#46570);
#4345=VERTEX_POINT('',#46629);
#4346=VERTEX_POINT('',#46648);
#4347=VERTEX_POINT('',#46650);
#4348=VERTEX_POINT('',#46669);
#5588=EDGE_CURVE('',#4305,#4305,#3472,.T.);
#5589=EDGE_CURVE('',#4305,#4306,#1331,.T.);
#5590=EDGE_CURVE('',#4307,#4306,#3473,.T.);
#5591=EDGE_CURVE('',#4308,#4307,#3474,.T.);
#5592=EDGE_CURVE('',#4306,#4308,#3475,.T.);
#5593=EDGE_CURVE('',#4309,#4310,#3476,.T.);
#5594=EDGE_CURVE('',#4309,#4311,#1332,.T.);
#5595=EDGE_CURVE('',#4311,#4312,#1333,.T.);
#5596=EDGE_CURVE('',#4312,#4313,#1334,.T.);
#5597=EDGE_CURVE('',#4313,#4314,#3477,.T.);
#5598=EDGE_CURVE('',#4314,#4315,#489,.T.);
#5599=EDGE_CURVE('',#4315,#4316,#490,.T.);
#5600=EDGE_CURVE('',#4317,#4316,#1335,.T.);
#5601=EDGE_CURVE('',#4317,#4318,#491,.T.);
#5602=EDGE_CURVE('',#4318,#4310,#492,.T.);
#5603=EDGE_CURVE('',#4319,#4320,#3478,.T.);
#5604=EDGE_CURVE('',#4320,#4321,#1336,.T.);
#5605=EDGE_CURVE('',#4321,#4321,#3479,.T.);
#5606=EDGE_CURVE('',#4320,#4322,#3480,.T.);
#5607=EDGE_CURVE('',#4322,#4319,#3481,.T.);
#5608=EDGE_CURVE('',#4323,#4324,#1337,.T.);
#5609=EDGE_CURVE('',#4324,#4325,#1338,.T.);
#5610=EDGE_CURVE('',#4325,#4326,#1339,.T.);
#5611=EDGE_CURVE('',#4326,#4323,#1340,.T.);
#5612=EDGE_CURVE('',#4327,#4328,#493,.T.);
#5613=EDGE_CURVE('',#4327,#4329,#494,.T.);
#5614=EDGE_CURVE('',#4329,#4330,#1341,.T.);
#5615=EDGE_CURVE('',#4330,#4331,#495,.T.);
#5616=EDGE_CURVE('',#4328,#4331,#1342,.T.);
#5617=EDGE_CURVE('',#4328,#4332,#3482,.T.);
#5618=EDGE_CURVE('',#4331,#4313,#3483,.T.);
#5619=EDGE_CURVE('',#4312,#4332,#496,.T.);
#5620=EDGE_CURVE('',#4333,#4334,#1343,.T.);
#5621=EDGE_CURVE('',#4334,#4335,#3484,.T.);
#5622=EDGE_CURVE('',#4335,#4336,#497,.T.);
#5623=EDGE_CURVE('',#4336,#4309,#3485,.T.);
#5624=EDGE_CURVE('',#4310,#4333,#498,.T.);
#5625=EDGE_CURVE('',#4330,#4337,#3486,.T.);
#5626=EDGE_CURVE('',#4337,#4338,#1344,.T.);
#5627=EDGE_CURVE('',#4338,#4314,#499,.T.);
#5628=EDGE_CURVE('',#4316,#4324,#500,.T.);
#5629=EDGE_CURVE('',#4323,#4317,#501,.T.);
#5630=EDGE_CURVE('',#4335,#4339,#1345,.T.);
#5631=EDGE_CURVE('',#4339,#4340,#502,.T.);
#5632=EDGE_CURVE('',#4340,#4341,#503,.T.);
#5633=EDGE_CURVE('',#4336,#4341,#1346,.T.);
#5634=EDGE_CURVE('',#4341,#4342,#3487,.T.);
#5635=EDGE_CURVE('',#4342,#4311,#504,.T.);
#5636=EDGE_CURVE('',#4340,#4307,#505,.T.);
#5637=EDGE_CURVE('',#4308,#4342,#506,.T.);
#5638=EDGE_CURVE('',#4332,#4322,#507,.T.);
#5639=EDGE_CURVE('',#4319,#4327,#508,.T.);
#5640=EDGE_CURVE('',#4311,#4343,#509,.T.);
#5641=EDGE_CURVE('',#4343,#4344,#510,.T.);
#5642=EDGE_CURVE('',#4344,#4345,#511,.T.);
#5643=EDGE_CURVE('',#4345,#4346,#1347,.T.);
#5644=EDGE_CURVE('',#4346,#4347,#512,.T.);
#5645=EDGE_CURVE('',#4347,#4348,#513,.T.);
#5646=EDGE_CURVE('',#4348,#4312,#121,.T.);
#5647=EDGE_CURVE('',#4324,#4338,#514,.T.);
#5648=EDGE_CURVE('',#4333,#4323,#515,.T.);
#5649=EDGE_CURVE('',#4325,#4337,#122,.T.);
#5650=EDGE_CURVE('',#4334,#4326,#123,.T.);
#5651=EDGE_CURVE('',#4329,#4346,#516,.T.);
#5652=EDGE_CURVE('',#4345,#4339,#517,.T.);
#5653=EDGE_CURVE('',#4307,#4344,#3488,.T.);
#5654=EDGE_CURVE('',#4308,#4343,#3489,.T.);
#5655=EDGE_CURVE('',#4347,#4319,#3490,.T.);
#5656=EDGE_CURVE('',#4348,#4322,#3491,.T.);
#8125=ORIENTED_EDGE('',*,*,#5588,.T.);
#8126=ORIENTED_EDGE('',*,*,#5589,.T.);
#8127=ORIENTED_EDGE('',*,*,#5590,.F.);
#8128=ORIENTED_EDGE('',*,*,#5591,.F.);
#8129=ORIENTED_EDGE('',*,*,#5592,.F.);
#8130=ORIENTED_EDGE('',*,*,#5589,.F.);
#8131=ORIENTED_EDGE('',*,*,#5593,.F.);
#8132=ORIENTED_EDGE('',*,*,#5594,.T.);
#8133=ORIENTED_EDGE('',*,*,#5595,.T.);
#8134=ORIENTED_EDGE('',*,*,#5596,.T.);
#8135=ORIENTED_EDGE('',*,*,#5597,.T.);
#8136=ORIENTED_EDGE('',*,*,#5598,.T.);
#8137=ORIENTED_EDGE('',*,*,#5599,.T.);
#8138=ORIENTED_EDGE('',*,*,#5600,.F.);
#8139=ORIENTED_EDGE('',*,*,#5601,.T.);
#8140=ORIENTED_EDGE('',*,*,#5602,.T.);
#8141=ORIENTED_EDGE('',*,*,#5603,.T.);
#8142=ORIENTED_EDGE('',*,*,#5604,.T.);
#8143=ORIENTED_EDGE('',*,*,#5605,.F.);
#8144=ORIENTED_EDGE('',*,*,#5604,.F.);
#8145=ORIENTED_EDGE('',*,*,#5606,.T.);
#8146=ORIENTED_EDGE('',*,*,#5607,.T.);
#8147=ORIENTED_EDGE('',*,*,#5608,.T.);
#8148=ORIENTED_EDGE('',*,*,#5609,.T.);
#8149=ORIENTED_EDGE('',*,*,#5610,.T.);
#8150=ORIENTED_EDGE('',*,*,#5611,.T.);
#8151=ORIENTED_EDGE('',*,*,#5612,.F.);
#8152=ORIENTED_EDGE('',*,*,#5613,.T.);
#8153=ORIENTED_EDGE('',*,*,#5614,.T.);
#8154=ORIENTED_EDGE('',*,*,#5615,.T.);
#8155=ORIENTED_EDGE('',*,*,#5616,.F.);
#8156=ORIENTED_EDGE('',*,*,#5617,.F.);
#8157=ORIENTED_EDGE('',*,*,#5616,.T.);
#8158=ORIENTED_EDGE('',*,*,#5618,.T.);
#8159=ORIENTED_EDGE('',*,*,#5596,.F.);
#8160=ORIENTED_EDGE('',*,*,#5619,.T.);
#8161=ORIENTED_EDGE('',*,*,#5620,.T.);
#8162=ORIENTED_EDGE('',*,*,#5621,.T.);
#8163=ORIENTED_EDGE('',*,*,#5622,.T.);
#8164=ORIENTED_EDGE('',*,*,#5623,.T.);
#8165=ORIENTED_EDGE('',*,*,#5593,.T.);
#8166=ORIENTED_EDGE('',*,*,#5624,.T.);
#8167=ORIENTED_EDGE('',*,*,#5588,.F.);
#8168=ORIENTED_EDGE('',*,*,#5615,.F.);
#8169=ORIENTED_EDGE('',*,*,#5625,.T.);
#8170=ORIENTED_EDGE('',*,*,#5626,.T.);
#8171=ORIENTED_EDGE('',*,*,#5627,.T.);
#8172=ORIENTED_EDGE('',*,*,#5597,.F.);
#8173=ORIENTED_EDGE('',*,*,#5618,.F.);
#8174=ORIENTED_EDGE('',*,*,#5605,.T.);
#8175=ORIENTED_EDGE('',*,*,#5600,.T.);
#8176=ORIENTED_EDGE('',*,*,#5628,.T.);
#8177=ORIENTED_EDGE('',*,*,#5608,.F.);
#8178=ORIENTED_EDGE('',*,*,#5629,.T.);
#8179=ORIENTED_EDGE('',*,*,#5622,.F.);
#8180=ORIENTED_EDGE('',*,*,#5630,.T.);
#8181=ORIENTED_EDGE('',*,*,#5631,.T.);
#8182=ORIENTED_EDGE('',*,*,#5632,.T.);
#8183=ORIENTED_EDGE('',*,*,#5633,.F.);
#8184=ORIENTED_EDGE('',*,*,#5633,.T.);
#8185=ORIENTED_EDGE('',*,*,#5634,.T.);
#8186=ORIENTED_EDGE('',*,*,#5635,.T.);
#8187=ORIENTED_EDGE('',*,*,#5594,.F.);
#8188=ORIENTED_EDGE('',*,*,#5623,.F.);
#8189=ORIENTED_EDGE('',*,*,#5632,.F.);
#8190=ORIENTED_EDGE('',*,*,#5636,.T.);
#8191=ORIENTED_EDGE('',*,*,#5590,.T.);
#8192=ORIENTED_EDGE('',*,*,#5592,.T.);
#8193=ORIENTED_EDGE('',*,*,#5637,.T.);
#8194=ORIENTED_EDGE('',*,*,#5634,.F.);
#8195=ORIENTED_EDGE('',*,*,#5617,.T.);
#8196=ORIENTED_EDGE('',*,*,#5638,.T.);
#8197=ORIENTED_EDGE('',*,*,#5606,.F.);
#8198=ORIENTED_EDGE('',*,*,#5603,.F.);
#8199=ORIENTED_EDGE('',*,*,#5639,.T.);
#8200=ORIENTED_EDGE('',*,*,#5612,.T.);
#8201=ORIENTED_EDGE('',*,*,#5595,.F.);
#8202=ORIENTED_EDGE('',*,*,#5640,.T.);
#8203=ORIENTED_EDGE('',*,*,#5641,.T.);
#8204=ORIENTED_EDGE('',*,*,#5642,.T.);
#8205=ORIENTED_EDGE('',*,*,#5643,.T.);
#8206=ORIENTED_EDGE('',*,*,#5644,.T.);
#8207=ORIENTED_EDGE('',*,*,#5645,.T.);
#8208=ORIENTED_EDGE('',*,*,#5646,.T.);
#8209=ORIENTED_EDGE('',*,*,#5598,.F.);
#8210=ORIENTED_EDGE('',*,*,#5627,.F.);
#8211=ORIENTED_EDGE('',*,*,#5647,.F.);
#8212=ORIENTED_EDGE('',*,*,#5628,.F.);
#8213=ORIENTED_EDGE('',*,*,#5599,.F.);
#8214=ORIENTED_EDGE('',*,*,#5601,.F.);
#8215=ORIENTED_EDGE('',*,*,#5629,.F.);
#8216=ORIENTED_EDGE('',*,*,#5648,.F.);
#8217=ORIENTED_EDGE('',*,*,#5624,.F.);
#8218=ORIENTED_EDGE('',*,*,#5602,.F.);
#8219=ORIENTED_EDGE('',*,*,#5647,.T.);
#8220=ORIENTED_EDGE('',*,*,#5626,.F.);
#8221=ORIENTED_EDGE('',*,*,#5649,.F.);
#8222=ORIENTED_EDGE('',*,*,#5609,.F.);
#8223=ORIENTED_EDGE('',*,*,#5648,.T.);
#8224=ORIENTED_EDGE('',*,*,#5611,.F.);
#8225=ORIENTED_EDGE('',*,*,#5650,.F.);
#8226=ORIENTED_EDGE('',*,*,#5620,.F.);
#8227=ORIENTED_EDGE('',*,*,#5614,.F.);
#8228=ORIENTED_EDGE('',*,*,#5651,.T.);
#8229=ORIENTED_EDGE('',*,*,#5643,.F.);
#8230=ORIENTED_EDGE('',*,*,#5652,.T.);
#8231=ORIENTED_EDGE('',*,*,#5630,.F.);
#8232=ORIENTED_EDGE('',*,*,#5621,.F.);
#8233=ORIENTED_EDGE('',*,*,#5650,.T.);
#8234=ORIENTED_EDGE('',*,*,#5610,.F.);
#8235=ORIENTED_EDGE('',*,*,#5649,.T.);
#8236=ORIENTED_EDGE('',*,*,#5625,.F.);
#8237=ORIENTED_EDGE('',*,*,#5652,.F.);
#8238=ORIENTED_EDGE('',*,*,#5642,.F.);
#8239=ORIENTED_EDGE('',*,*,#5653,.F.);
#8240=ORIENTED_EDGE('',*,*,#5636,.F.);
#8241=ORIENTED_EDGE('',*,*,#5631,.F.);
#8242=ORIENTED_EDGE('',*,*,#5653,.T.);
#8243=ORIENTED_EDGE('',*,*,#5641,.F.);
#8244=ORIENTED_EDGE('',*,*,#5654,.F.);
#8245=ORIENTED_EDGE('',*,*,#5591,.T.);
#8246=ORIENTED_EDGE('',*,*,#5635,.F.);
#8247=ORIENTED_EDGE('',*,*,#5637,.F.);
#8248=ORIENTED_EDGE('',*,*,#5654,.T.);
#8249=ORIENTED_EDGE('',*,*,#5640,.F.);
#8250=ORIENTED_EDGE('',*,*,#5613,.F.);
#8251=ORIENTED_EDGE('',*,*,#5639,.F.);
#8252=ORIENTED_EDGE('',*,*,#5655,.F.);
#8253=ORIENTED_EDGE('',*,*,#5644,.F.);
#8254=ORIENTED_EDGE('',*,*,#5651,.F.);
#8255=ORIENTED_EDGE('',*,*,#5655,.T.);
#8256=ORIENTED_EDGE('',*,*,#5607,.F.);
#8257=ORIENTED_EDGE('',*,*,#5656,.F.);
#8258=ORIENTED_EDGE('',*,*,#5645,.F.);
#8259=ORIENTED_EDGE('',*,*,#5619,.F.);
#8260=ORIENTED_EDGE('',*,*,#5646,.F.);
#8261=ORIENTED_EDGE('',*,*,#5656,.T.);
#8262=ORIENTED_EDGE('',*,*,#5638,.F.);
#8868=ADVANCED_FACE('',(#2518),#2042,.F.);
#8869=ADVANCED_FACE('',(#2519),#2043,.T.);
#8870=ADVANCED_FACE('',(#2520),#2044,.F.);
#8871=ADVANCED_FACE('',(#2521),#873,.F.);
#8872=ADVANCED_FACE('',(#2522),#133,.F.);
#8873=ADVANCED_FACE('',(#2523),#2045,.F.);
#8874=ADVANCED_FACE('',(#2524,#753),#874,.F.);
#8875=ADVANCED_FACE('',(#2525,#754),#875,.T.);
#8876=ADVANCED_FACE('',(#2526),#134,.F.);
#8877=ADVANCED_FACE('',(#2527),#135,.F.);
#8878=ADVANCED_FACE('',(#2528),#2046,.F.);
#8879=ADVANCED_FACE('',(#2529),#876,.T.);
#8880=ADVANCED_FACE('',(#2530),#877,.F.);
#8881=ADVANCED_FACE('',(#2531),#136,.T.);
#8882=ADVANCED_FACE('',(#2532),#598,.T.);
#8883=ADVANCED_FACE('',(#2533),#599,.T.);
#8884=ADVANCED_FACE('',(#2534),#2047,.T.);
#8885=ADVANCED_FACE('',(#2535),#2048,.T.);
#8886=ADVANCED_FACE('',(#2536),#2049,.T.);
#8887=ADVANCED_FACE('',(#2537),#600,.F.);
#8888=ADVANCED_FACE('',(#2538),#601,.F.);
#8889=ADVANCED_FACE('',(#2539),#602,.F.);
#8890=ADVANCED_FACE('',(#2540),#603,.F.);
#8891=ADVANCED_FACE('',(#2541),#604,.F.);
#8892=ADVANCED_FACE('',(#2542),#605,.F.);
#8935=CLOSED_SHELL('',(#8868,#8869,#8870,#8871,#8872,#8873,#8874,#8875,
#8876,#8877,#8878,#8879,#8880,#8881,#8882,#8883,#8884,#8885,#8886,#8887,
#8888,#8889,#8890,#8891,#8892));
#9834=AXIS2_PLACEMENT_3D('',#45932,#11932,#11933);
#9835=AXIS2_PLACEMENT_3D('',#45933,#11934,#11935);
#9836=AXIS2_PLACEMENT_3D('',#45935,#11936,#11937);
#9837=AXIS2_PLACEMENT_3D('',#45939,#11939,#11940);
#9838=AXIS2_PLACEMENT_3D('',#45941,#11941,#11942);
#9839=AXIS2_PLACEMENT_3D('',#45942,#11943,#11944);
#9840=AXIS2_PLACEMENT_3D('',#45943,#11945,#11946);
#9841=AXIS2_PLACEMENT_3D('',#45946,#11947,#11948);
#9842=AXIS2_PLACEMENT_3D('',#45954,#11952,#11953);
#9843=AXIS2_PLACEMENT_3D('',#46082,#11955,#11956);
#9844=AXIS2_PLACEMENT_3D('',#46085,#11957,#11958);
#9845=AXIS2_PLACEMENT_3D('',#46088,#11960,#11961);
#9846=AXIS2_PLACEMENT_3D('',#46090,#11962,#11963);
#9847=AXIS2_PLACEMENT_3D('',#46091,#11964,#11965);
#9848=AXIS2_PLACEMENT_3D('',#46092,#11966,#11967);
#9849=AXIS2_PLACEMENT_3D('',#46138,#11974,#11975);
#9850=AXIS2_PLACEMENT_3D('',#46140,#11976,#11977);
#9851=AXIS2_PLACEMENT_3D('',#46141,#11978,#11979);
#9852=AXIS2_PLACEMENT_3D('',#46154,#11980,#11981);
#9853=AXIS2_PLACEMENT_3D('',#46159,#11983,#11984);
#9854=AXIS2_PLACEMENT_3D('',#46167,#11985,#11986);
#9855=AXIS2_PLACEMENT_3D('',#46247,#11987,#11988);
#9856=AXIS2_PLACEMENT_3D('',#46249,#11989,#11990);
#9857=AXIS2_PLACEMENT_3D('',#46414,#11994,#11995);
#9858=AXIS2_PLACEMENT_3D('',#46416,#11996,#11997);
#9859=AXIS2_PLACEMENT_3D('',#46429,#11998,#11999);
#9860=AXIS2_PLACEMENT_3D('',#46471,#12000,#12001);
#9861=AXIS2_PLACEMENT_3D('',#46725,#12003,#12004);
#9862=AXIS2_PLACEMENT_3D('',#47028,#12005,#12006);
#9863=AXIS2_PLACEMENT_3D('',#47029,#12007,#12008);
#9864=AXIS2_PLACEMENT_3D('',#47030,#12009,#12010);
#9865=AXIS2_PLACEMENT_3D('',#47031,#12011,#12012);
#9866=AXIS2_PLACEMENT_3D('',#47032,#12013,#12014);
#9867=AXIS2_PLACEMENT_3D('',#47139,#12015,#12016);
#9868=AXIS2_PLACEMENT_3D('',#47206,#12017,#12018);
#9869=AXIS2_PLACEMENT_3D('',#47309,#12019,#12020);
#9870=AXIS2_PLACEMENT_3D('',#47376,#12021,#12022);
#11932=DIRECTION('axis',(0.,0.,1.));
#11933=DIRECTION('refdir',(1.,0.,0.));
#11934=DIRECTION('center_axis',(4.00051694051949E-18,-1.90113600208472E-18,
-1.));
#11935=DIRECTION('ref_axis',(-0.348963627142735,-0.937136269136664,3.85588598105426E-19));
#11936=DIRECTION('center_axis',(-4.00051694051949E-18,1.90113600208472E-18,
1.));
#11937=DIRECTION('ref_axis',(0.348963627142735,0.937136269136664,-3.85588598105426E-19));
#11938=DIRECTION('',(4.00051694051949E-18,-1.90113600208472E-18,-1.));
#11939=DIRECTION('center_axis',(-4.00051694051949E-18,1.90113600208472E-18,
1.));
#11940=DIRECTION('ref_axis',(-0.348963627142721,-0.93713626913667,3.85588598105494E-19));
#11941=DIRECTION('center_axis',(-4.00051694051949E-18,1.90113600208472E-18,
1.));
#11942=DIRECTION('ref_axis',(-0.348963627142735,-0.937136269136664,3.85588598105426E-19));
#11943=DIRECTION('center_axis',(-4.00051694051949E-18,1.90113600208472E-18,
1.));
#11944=DIRECTION('ref_axis',(-0.348963627142721,-0.93713626913667,3.85588598105494E-19));
#11945=DIRECTION('center_axis',(4.00051694051949E-18,-1.90113600208472E-18,
-1.));
#11946=DIRECTION('ref_axis',(-0.587778313469371,0.809022035679562,-3.88947801881448E-18));
#11947=DIRECTION('center_axis',(-4.00051694051949E-18,1.90113600208472E-18,
1.));
#11948=DIRECTION('ref_axis',(-0.348963627142725,-0.937136269136668,3.85588598105472E-19));
#11949=DIRECTION('',(4.0005169405195E-18,-1.90113600208472E-18,-1.));
#11950=DIRECTION('',(0.,0.,-1.));
#11951=DIRECTION('',(4.0005169405195E-18,-1.90113600208472E-18,-1.));
#11952=DIRECTION('center_axis',(-4.00051694051949E-18,1.90113600208472E-18,
1.));
#11953=DIRECTION('ref_axis',(-0.348963627142725,-0.937136269136668,3.85588598105472E-19));
#11954=DIRECTION('',(4.0005169405195E-18,-1.90113600208472E-18,-1.));
#11955=DIRECTION('center_axis',(4.00051694051949E-18,-1.90113600208472E-18,
-1.));
#11956=DIRECTION('ref_axis',(-0.348963627142735,-0.937136269136664,3.85588598105426E-19));
#11957=DIRECTION('center_axis',(-4.00051694051949E-18,1.90113600208472E-18,
1.));
#11958=DIRECTION('ref_axis',(-0.348963627142721,-0.93713626913667,3.85588598105494E-19));
#11959=DIRECTION('',(4.00051694051949E-18,-1.90113600208472E-18,-1.));
#11960=DIRECTION('center_axis',(-4.00051694051949E-18,1.90113600208472E-18,
1.));
#11961=DIRECTION('ref_axis',(0.348963627142735,0.937136269136664,-3.85588598105426E-19));
#11962=DIRECTION('center_axis',(-4.00051694051949E-18,1.90113600208472E-18,
1.));
#11963=DIRECTION('ref_axis',(-0.348963627142721,-0.93713626913667,3.85588598105494E-19));
#11964=DIRECTION('center_axis',(-4.00051694051949E-18,1.90113600208472E-18,
1.));
#11965=DIRECTION('ref_axis',(-0.348963627142735,-0.937136269136664,3.85588598105426E-19));
#11966=DIRECTION('center_axis',(0.348963627142731,0.937136269136666,-3.85588598105444E-19));
#11967=DIRECTION('ref_axis',(4.00051694051949E-18,-1.90113600208472E-18,
-1.));
#11968=DIRECTION('',(4.0005169405195E-18,-1.90113600208472E-18,-1.));
#11969=DIRECTION('',(0.937136269136666,-0.348963627142731,4.41245683523558E-18));
#11970=DIRECTION('',(-4.0005169405195E-18,1.90113600208472E-18,1.));
#11971=DIRECTION('',(-0.937136269136666,0.348963627142731,-4.41245683523558E-18));
#11972=DIRECTION('',(4.0005169405195E-18,-1.90113600208472E-18,-1.));
#11973=DIRECTION('',(4.0005169405195E-18,-1.90113600208472E-18,-1.));
#11974=DIRECTION('center_axis',(4.00051694051949E-18,-1.90113600208472E-18,
-1.));
#11975=DIRECTION('ref_axis',(-0.348963627142731,-0.937136269136666,3.85588598105444E-19));
#11976=DIRECTION('center_axis',(4.00051694051949E-18,-1.90113600208472E-18,
-1.));
#11977=DIRECTION('ref_axis',(-0.348963627142731,-0.937136269136666,3.85588598105444E-19));
#11978=DIRECTION('center_axis',(4.00051694051949E-18,-1.90113600208472E-18,
-1.));
#11979=DIRECTION('ref_axis',(-0.348963627142731,-0.937136269136666,3.85588598105444E-19));
#11980=DIRECTION('center_axis',(4.00051694051949E-18,-1.90113600208472E-18,
-1.));
#11981=DIRECTION('ref_axis',(-0.348963627142731,-0.937136269136666,3.85588598105444E-19));
#11982=DIRECTION('',(0.937136269136666,-0.348963627142731,4.41245683523558E-18));
#11983=DIRECTION('center_axis',(-4.00051694051949E-18,1.90113600208472E-18,
1.));
#11984=DIRECTION('ref_axis',(-0.348963627142846,-0.937136269136623,3.85588598104903E-19));
#11985=DIRECTION('center_axis',(4.00051694051949E-18,-1.90113600208472E-18,
-1.));
#11986=DIRECTION('ref_axis',(-0.348963627142731,-0.937136269136666,3.85588598105444E-19));
#11987=DIRECTION('center_axis',(4.00051694051949E-18,-1.90113600208472E-18,
-1.));
#11988=DIRECTION('ref_axis',(-0.348963627142731,-0.937136269136666,3.85588598105444E-19));
#11989=DIRECTION('center_axis',(4.00051694051949E-18,-1.90113600208472E-18,
-1.));
#11990=DIRECTION('ref_axis',(-0.348963627142735,-0.937136269136664,3.85588598105426E-19));
#11991=DIRECTION('',(-0.937136269136666,0.348963627142731,-4.41245683523558E-18));
#11992=DIRECTION('',(4.0005169405195E-18,-1.90113600208472E-18,-1.));
#11993=DIRECTION('',(4.0005169405195E-18,-1.90113600208472E-18,-1.));
#11994=DIRECTION('center_axis',(4.00051694051949E-18,-1.90113600208472E-18,
-1.));
#11995=DIRECTION('ref_axis',(-0.348963627142731,-0.937136269136666,3.85588598105444E-19));
#11996=DIRECTION('center_axis',(4.00051694051949E-18,-1.90113600208472E-18,
-1.));
#11997=DIRECTION('ref_axis',(-0.348963627142731,-0.937136269136666,3.85588598105444E-19));
#11998=DIRECTION('center_axis',(4.00051694051949E-18,-1.90113600208472E-18,
-1.));
#11999=DIRECTION('ref_axis',(-0.348963627142731,-0.937136269136666,3.85588598105444E-19));
#12000=DIRECTION('center_axis',(4.00051694051949E-18,-1.90113600208472E-18,
-1.));
#12001=DIRECTION('ref_axis',(-0.348963627142731,-0.937136269136666,3.85588598105444E-19));
#12002=DIRECTION('',(4.0005169405195E-18,-1.90113600208472E-18,-1.));
#12003=DIRECTION('center_axis',(0.,0.,-1.));
#12004=DIRECTION('ref_axis',(-0.125309381306763,0.992117714264046,0.));
#12005=DIRECTION('center_axis',(-0.937136269136666,0.348963627142731,-4.41245683523558E-18));
#12006=DIRECTION('ref_axis',(-4.13507333629925E-18,1.53978694183454E-18,
1.));
#12007=DIRECTION('center_axis',(0.662655410802406,-0.246754547140085,0.707106781186538));
#12008=DIRECTION('ref_axis',(0.66265541080291,-0.246754547138675,-0.707106781186557));
#12009=DIRECTION('center_axis',(0.937136269136666,-0.348963627142731,4.41245683523558E-18));
#12010=DIRECTION('ref_axis',(4.13507333629925E-18,-1.53978694183454E-18,
-1.));
#12011=DIRECTION('center_axis',(0.662655410802405,-0.246754547140073,-0.707106781186543));
#12012=DIRECTION('ref_axis',(0.662655410801971,-0.246754547141213,0.707106781186552));
#12013=DIRECTION('center_axis',(4.00051694051949E-18,-1.90113600208472E-18,
-1.));
#12014=DIRECTION('ref_axis',(-0.348963627142735,-0.937136269136664,3.85588598105426E-19));
#12015=DIRECTION('center_axis',(-0.352532537381825,-0.935799556575623,3.68769839860518E-19));
#12016=DIRECTION('ref_axis',(0.935799556575623,-0.352532537381825,6.00067969352728E-34));
#12017=DIRECTION('center_axis',(-0.362140169981158,-0.932123649139972,2.90655021385084E-12));
#12018=DIRECTION('ref_axis',(0.932123649139972,-0.362140169981158,-2.43759966809478E-27));
#12019=DIRECTION('center_axis',(-0.352532537381905,-0.935799556575593,3.46813776064964E-15));
#12020=DIRECTION('ref_axis',(0.935799556575593,-0.352532537381904,-3.73856855277001E-30));
#12021=DIRECTION('center_axis',(-0.362140169981175,-0.932123649139966,-2.71107876657752E-13));
#12022=DIRECTION('ref_axis',(0.932123649139966,-0.362140169981175,-1.23386467665282E-27));
#45932=CARTESIAN_POINT('',(0.,0.,0.));
#45933=CARTESIAN_POINT('Origin',(-84.8548278771908,-59.0746191263193,178.585485069079));
#45934=CARTESIAN_POINT('',(-84.5058642500481,-58.1374828571826,178.585485069079));
#45935=CARTESIAN_POINT('Origin',(-84.8548278771908,-59.0746191263193,178.585485069079));
#45936=CARTESIAN_POINT('',(-84.5058642500481,-58.1374828571826,177.685485069079));
#45937=CARTESIAN_POINT('',(-84.5058642500481,-58.1374828571826,178.585485069079));
#45938=CARTESIAN_POINT('',(-85.5577653075767,-59.7858708180308,177.685485069079));
#45939=CARTESIAN_POINT('Origin',(-84.8548278771908,-59.0746191263193,177.685485069079));
#45940=CARTESIAN_POINT('',(-84.9035795890701,-58.0758081979705,177.685485069079));
#45941=CARTESIAN_POINT('Origin',(-84.8548278771908,-59.0746191263193,177.685485069079));
#45942=CARTESIAN_POINT('Origin',(-84.8548278771908,-59.0746191263193,177.685485069079));
#45943=CARTESIAN_POINT('Origin',(-77.596384432622,-39.5821847282766,178.585485069079));
#45944=CARTESIAN_POINT('',(-77.03410267114,-39.7915629045623,178.585485069079));
#45945=CARTESIAN_POINT('',(-77.4650015118991,-40.1676234767637,178.585484926558));
#45946=CARTESIAN_POINT('Origin',(-77.596384432622,-39.5821847282766,178.585485069079));
#45947=CARTESIAN_POINT('',(-77.2498704957138,-39.7773398653825,177.055074234203));
#45948=CARTESIAN_POINT('',(-77.03410267114,-39.7915629045623,178.585485069079));
#45949=CARTESIAN_POINT('',(-77.2498571612849,-39.7773460826798,174.915920053832));
#45950=CARTESIAN_POINT('',(-77.3304501603129,-39.7397688129298,177.185345426401));
#45951=CARTESIAN_POINT('',(-77.03410267114,-39.7915629045623,173.385485069079));
#45952=CARTESIAN_POINT('',(-77.03410267114,-39.7915629045623,178.585485069079));
#45953=CARTESIAN_POINT('',(-77.4650015118991,-40.1676234767637,173.3854852116));
#45954=CARTESIAN_POINT('Origin',(-77.596384432622,-39.5821847282766,173.385485069079));
#45955=CARTESIAN_POINT('',(-77.8056987826698,-40.1445035064164,173.433770774959));
#45956=CARTESIAN_POINT('Ctrl Pts',(-77.4650015118379,-40.167623476675,173.385485354513));
#45957=CARTESIAN_POINT('Ctrl Pts',(-77.5222920678253,-40.1804805015978,
173.385517889895));
#45958=CARTESIAN_POINT('Ctrl Pts',(-77.580890468835,-40.1848056038886,173.38835249126));
#45959=CARTESIAN_POINT('Ctrl Pts',(-77.6971422272215,-40.1765308873483,
173.403655693534));
#45960=CARTESIAN_POINT('Ctrl Pts',(-77.7531232269699,-40.1640606597343,
173.415935467735));
#45961=CARTESIAN_POINT('Ctrl Pts',(-77.8056942667798,-40.1444919337478,
173.433771387659));
#45962=CARTESIAN_POINT('',(-78.1586259806643,-39.3728300600142,174.385485069105));
#45963=CARTESIAN_POINT('Ctrl Pts',(-77.8056987826698,-40.1445035064164,
173.433770774959));
#45964=CARTESIAN_POINT('Ctrl Pts',(-77.8316025753951,-40.1348599999348,
173.442559365324));
#45965=CARTESIAN_POINT('Ctrl Pts',(-77.8563162910818,-40.1235859591036,
173.452576825659));
#45966=CARTESIAN_POINT('Ctrl Pts',(-77.8797393924345,-40.110999573227,173.463759860592));
#45967=CARTESIAN_POINT('Ctrl Pts',(-77.9021524569635,-40.0989559298771,
173.474460667449));
#45968=CARTESIAN_POINT('Ctrl Pts',(-77.9233830575993,-40.0857111079833,
173.486228127983));
#45969=CARTESIAN_POINT('Ctrl Pts',(-77.9433549726383,-40.071538020758,173.498955663141));
#45970=CARTESIAN_POINT('Ctrl Pts',(-77.9633241715251,-40.0573668610525,
173.511681467373));
#45971=CARTESIAN_POINT('Ctrl Pts',(-77.982034331596,-40.0422680834381,173.525366622401));
#45972=CARTESIAN_POINT('Ctrl Pts',(-77.9994322577124,-40.0265023515187,
173.539859446119));
#45973=CARTESIAN_POINT('Ctrl Pts',(-78.0169241204228,-40.0106514957089,
173.554430520915));
#45974=CARTESIAN_POINT('Ctrl Pts',(-78.0330889895565,-39.9941267838722,
173.569817339963));
#45975=CARTESIAN_POINT('Ctrl Pts',(-78.047905558146,-39.9771754028481,173.585828643786));
#45976=CARTESIAN_POINT('Ctrl Pts',(-78.049822621609,-39.9749821235464,173.58790028982));
#45977=CARTESIAN_POINT('Ctrl Pts',(-78.0517171641965,-39.9727816736662,
173.589982348299));
#45978=CARTESIAN_POINT('Ctrl Pts',(-78.0535891860334,-39.9705745632887,
173.592074369728));
#45979=CARTESIAN_POINT('Ctrl Pts',(-78.0728330194838,-39.9478861182751,
173.613579734231));
#45980=CARTESIAN_POINT('Ctrl Pts',(-78.089853382054,-39.924453320363,173.636258615212));
#45981=CARTESIAN_POINT('Ctrl Pts',(-78.1047842555492,-39.9005911821429,
173.659865265467));
#45982=CARTESIAN_POINT('Ctrl Pts',(-78.1206592741246,-39.875220135525,173.684964668486));
#45983=CARTESIAN_POINT('Ctrl Pts',(-78.1341726700168,-39.8493634840486,
173.711112013678));
#45984=CARTESIAN_POINT('Ctrl Pts',(-78.1455328604065,-39.8233751616464,
173.738044096303));
#45985=CARTESIAN_POINT('Ctrl Pts',(-78.1568930507962,-39.7973868392441,
173.764976178928));
#45986=CARTESIAN_POINT('Ctrl Pts',(-78.1661010214841,-39.7712663408389,
173.792692834852));
#45987=CARTESIAN_POINT('Ctrl Pts',(-78.1733990074322,-39.7453499152769,
173.820969559096));
#45988=CARTESIAN_POINT('Ctrl Pts',(-78.18109670286,-39.7180140513866,173.850794994835));
#45989=CARTESIAN_POINT('Ctrl Pts',(-78.1866425628593,-39.6907966187179,
173.881282707479));
#45990=CARTESIAN_POINT('Ctrl Pts',(-78.1902997744162,-39.6639645935433,
173.912302936584));
#45991=CARTESIAN_POINT('Ctrl Pts',(-78.1942435916019,-39.6350298162232,
173.945754135879));
#45992=CARTESIAN_POINT('Ctrl Pts',(-78.1959924060582,-39.6065425527247,
173.979825829551));
#45993=CARTESIAN_POINT('Ctrl Pts',(-78.1958486262586,-39.5788540211706,
174.014408581675));
#45994=CARTESIAN_POINT('Ctrl Pts',(-78.1957540319387,-39.5606374301254,
174.037160956659));
#45995=CARTESIAN_POINT('Ctrl Pts',(-78.194839549217,-39.5427669704748,174.060135624983));
#45996=CARTESIAN_POINT('Ctrl Pts',(-78.1931823226566,-39.5253477403486,
174.083307866194));
#45997=CARTESIAN_POINT('Ctrl Pts',(-78.1917910998975,-39.5107244957194,
174.102760697886));
#45998=CARTESIAN_POINT('Ctrl Pts',(-78.1898418665052,-39.4963423543713,
174.122368986697));
#45999=CARTESIAN_POINT('Ctrl Pts',(-78.1874866612736,-39.4823936898877,
174.142301808365));
#46000=CARTESIAN_POINT('Ctrl Pts',(-78.1851541826915,-39.4685796236137,
174.162042287453));
#46001=CARTESIAN_POINT('Ctrl Pts',(-78.1824234178568,-39.4551907750551,
174.182101870072));
#46002=CARTESIAN_POINT('Ctrl Pts',(-78.1793987895934,-39.4424389285065,
174.202635548891));
#46003=CARTESIAN_POINT('Ctrl Pts',(-78.1783297262753,-39.4379317526833,
174.209893235091));
#46004=CARTESIAN_POINT('Ctrl Pts',(-78.1772235617853,-39.4335043809312,
174.21721000765));
#46005=CARTESIAN_POINT('Ctrl Pts',(-78.1760836397663,-39.4291668947634,
174.224592137249));
#46006=CARTESIAN_POINT('Ctrl Pts',(-78.1730777137475,-39.4177291276969,
174.244058499917));
#46007=CARTESIAN_POINT('Ctrl Pts',(-78.1696683952291,-39.4065841791719,
174.264097692483));
#46008=CARTESIAN_POINT('Ctrl Pts',(-78.1666558229229,-39.397272372026,174.284826885168));
#46009=CARTESIAN_POINT('Ctrl Pts',(-78.1637494748364,-39.3882889020444,
174.304825160187));
#46010=CARTESIAN_POINT('Ctrl Pts',(-78.1612120338452,-39.3810116904671,
174.325466196324));
#46011=CARTESIAN_POINT('Ctrl Pts',(-78.1597309734151,-39.3768406404591,
174.346822553575));
#46012=CARTESIAN_POINT('Ctrl Pts',(-78.1588547323164,-39.3743729184355,
174.359457634198));
#46013=CARTESIAN_POINT('Ctrl Pts',(-78.1583476777879,-39.3729927506605,
174.372342435271));
#46014=CARTESIAN_POINT('Ctrl Pts',(-78.1583476777881,-39.3729927506605,
174.385485069047));
#46015=CARTESIAN_POINT('',(-78.1586244653881,-39.3728309458164,177.585485069077));
#46016=CARTESIAN_POINT('',(-78.158666194104,-39.372806551991,178.585485069079));
#46017=CARTESIAN_POINT('',(-77.8056988610362,-40.1445034772439,178.537199336601));
#46018=CARTESIAN_POINT('Ctrl Pts',(-78.1583476777881,-39.3729927506604,
177.585485069082));
#46019=CARTESIAN_POINT('Ctrl Pts',(-78.1583476777881,-39.3729927506605,
177.606543111377));
#46020=CARTESIAN_POINT('Ctrl Pts',(-78.1596294469341,-39.3764978870272,
177.626857265634));
#46021=CARTESIAN_POINT('Ctrl Pts',(-78.1616381613638,-39.3823135423054,
177.646497387667));
#46022=CARTESIAN_POINT('Ctrl Pts',(-78.1637229995436,-39.3883495920224,
177.666881806511));
#46023=CARTESIAN_POINT('Ctrl Pts',(-78.1665913487967,-39.3968744879276,
177.686540737803));
#46024=CARTESIAN_POINT('Ctrl Pts',(-78.1695883704607,-39.4065726866962,
177.705593053786));
#46025=CARTESIAN_POINT('Ctrl Pts',(-78.1717716424418,-39.4136376358397,
177.719472295355));
#46026=CARTESIAN_POINT('Ctrl Pts',(-78.174022450919,-39.4213256630031,177.733030512162));
#46027=CARTESIAN_POINT('Ctrl Pts',(-78.1760752475433,-39.4291349653113,
177.746323654485));
#46028=CARTESIAN_POINT('Ctrl Pts',(-78.1796664380935,-39.4427966658032,
177.769578859858));
#46029=CARTESIAN_POINT('Ctrl Pts',(-78.1829591937475,-39.4574596072776,
177.792348582069));
#46030=CARTESIAN_POINT('Ctrl Pts',(-78.1857889481807,-39.4727725746961,
177.814748829435));
#46031=CARTESIAN_POINT('Ctrl Pts',(-78.1886413594616,-39.4882081476548,
177.837328427697));
#46032=CARTESIAN_POINT('Ctrl Pts',(-78.1910235140542,-39.5043040816822,
177.859533548057));
#46033=CARTESIAN_POINT('Ctrl Pts',(-78.1927230572288,-39.520725590416,177.881497529369));
#46034=CARTESIAN_POINT('Ctrl Pts',(-78.1928989309815,-39.5224249366932,
177.883770427096));
#46035=CARTESIAN_POINT('Ctrl Pts',(-78.1930674551391,-39.5241277921344,
177.886040747814));
#46036=CARTESIAN_POINT('Ctrl Pts',(-78.1932283667941,-39.5258338015101,
177.888308641737));
#46037=CARTESIAN_POINT('Ctrl Pts',(-78.1951412252173,-39.5461142119357,
177.915268528484));
#46038=CARTESIAN_POINT('Ctrl Pts',(-78.1960338984988,-39.5668410266997,
177.941748603447));
#46039=CARTESIAN_POINT('Ctrl Pts',(-78.1958302050792,-39.5879108654907,
177.967815585286));
#46040=CARTESIAN_POINT('Ctrl Pts',(-78.1956284950027,-39.6087755493006,
177.993628755446));
#46041=CARTESIAN_POINT('Ctrl Pts',(-78.1943515214607,-39.6299766883225,
178.0190380862));
#46042=CARTESIAN_POINT('Ctrl Pts',(-78.1918820718927,-39.6514390060816,
178.044100477535));
#46043=CARTESIAN_POINT('Ctrl Pts',(-78.1894808174157,-39.6723086311488,
178.068470758337));
#46044=CARTESIAN_POINT('Ctrl Pts',(-78.1859515928356,-39.6934254635894,
178.092514045181));
#46045=CARTESIAN_POINT('Ctrl Pts',(-78.181150111863,-39.7147415708539,178.116258460794));
#46046=CARTESIAN_POINT('Ctrl Pts',(-78.1788875895975,-39.7247860066383,
178.127447148058));
#46047=CARTESIAN_POINT('Ctrl Pts',(-78.176342078521,-39.7348749783378,178.138569023899));
#46048=CARTESIAN_POINT('Ctrl Pts',(-78.1734960538477,-39.7450048916319,
178.149624088881));
#46049=CARTESIAN_POINT('Ctrl Pts',(-78.1664823260289,-39.7699689951893,
178.176868131256));
#46050=CARTESIAN_POINT('Ctrl Pts',(-78.1577095484763,-39.7951364254273,
178.203590494714));
#46051=CARTESIAN_POINT('Ctrl Pts',(-78.1469244962564,-39.8202256160684,
178.229632583319));
#46052=CARTESIAN_POINT('Ctrl Pts',(-78.1365609419034,-39.8443342792052,
178.254656903574));
#46053=CARTESIAN_POINT('Ctrl Pts',(-78.1243384322505,-39.8683711781007,
178.279053143627));
#46054=CARTESIAN_POINT('Ctrl Pts',(-78.1100449468631,-39.8920804832296,
178.302635096528));
#46055=CARTESIAN_POINT('Ctrl Pts',(-78.0964140060138,-39.9146907932435,
178.325123957459));
#46056=CARTESIAN_POINT('Ctrl Pts',(-78.0808988659364,-39.9370035953691,
178.346871943661));
#46057=CARTESIAN_POINT('Ctrl Pts',(-78.0633391929321,-39.9587850372975,
178.367677462424));
#46058=CARTESIAN_POINT('Ctrl Pts',(-78.0600909570606,-39.962814227419,178.371526123636));
#46059=CARTESIAN_POINT('Ctrl Pts',(-78.0567728460438,-39.9668251906836,
178.375342428917));
#46060=CARTESIAN_POINT('Ctrl Pts',(-78.0533839713637,-39.9708163811803,
178.37912496045));
#46061=CARTESIAN_POINT('Ctrl Pts',(-78.0381562345498,-39.9887505936238,
178.3961215744));
#46062=CARTESIAN_POINT('Ctrl Pts',(-78.0214792509514,-40.0061786390317,
178.412402159754));
#46063=CARTESIAN_POINT('Ctrl Pts',(-78.0034060666603,-40.0228415926461,
178.427758408585));
#46064=CARTESIAN_POINT('Ctrl Pts',(-77.9862521315262,-40.0386570251032,
178.442333598662));
#46065=CARTESIAN_POINT('Ctrl Pts',(-77.9678413089092,-40.0537827074521,
178.45607577319));
#46066=CARTESIAN_POINT('Ctrl Pts',(-77.9482495099567,-40.0679806950435,
178.468847266813));
#46067=CARTESIAN_POINT('Ctrl Pts',(-77.928632010329,-40.0821973076662,178.481635514181));
#46068=CARTESIAN_POINT('Ctrl Pts',(-77.9078311666701,-40.0954833749289,
178.493450152086));
#46069=CARTESIAN_POINT('Ctrl Pts',(-77.8859429696398,-40.1075895985258,
178.504200235491));
#46070=CARTESIAN_POINT('Ctrl Pts',(-77.8638991823429,-40.1197818781168,
178.51502673489));
#46071=CARTESIAN_POINT('Ctrl Pts',(-77.8407533339131,-40.130777031073,178.524773356882));
#46072=CARTESIAN_POINT('Ctrl Pts',(-77.8166118463901,-40.1403164142105,
178.533399105501));
#46073=CARTESIAN_POINT('Ctrl Pts',(-77.8129963943436,-40.1417450412681,
178.534690905787));
#46074=CARTESIAN_POINT('Ctrl Pts',(-77.8093586138701,-40.1431410178554,
178.535957662038));
#46075=CARTESIAN_POINT('Ctrl Pts',(-77.8056988610362,-40.1445034772439,
178.537199336601));
#46076=CARTESIAN_POINT('Ctrl Pts',(-77.8056943451453,-40.1444919045775,
178.537198723902));
#46077=CARTESIAN_POINT('Ctrl Pts',(-77.7534354935633,-40.1639444317979,
178.554928733475));
#46078=CARTESIAN_POINT('Ctrl Pts',(-77.6978009243969,-40.1763845824508,
178.567170792542));
#46079=CARTESIAN_POINT('Ctrl Pts',(-77.5815770850698,-40.1848554744716,
178.582583818994));
#46080=CARTESIAN_POINT('Ctrl Pts',(-77.5226296507783,-40.1805562612473,
178.585452056548));
#46081=CARTESIAN_POINT('Ctrl Pts',(-77.4650015118378,-40.167623476675,178.585484783646));
#46082=CARTESIAN_POINT('Origin',(-84.8548278771908,-59.0746191263193,178.585485069079));
#46083=CARTESIAN_POINT('',(-85.5577653075812,-59.7858708180264,174.285485069079));
#46084=CARTESIAN_POINT('',(-84.5058642500481,-58.1374828571826,174.285485069079));
#46085=CARTESIAN_POINT('Origin',(-84.8548278771908,-59.0746191263193,174.285485069079));
#46086=CARTESIAN_POINT('',(-84.5058642500481,-58.1374828571826,173.385485069079));
#46087=CARTESIAN_POINT('',(-84.5058642500481,-58.1374828571826,178.585485069079));
#46088=CARTESIAN_POINT('Origin',(-84.8548278771908,-59.0746191263193,173.385485069079));
#46089=CARTESIAN_POINT('',(-84.9035795890703,-58.0758081979706,174.285485069079));
#46090=CARTESIAN_POINT('Origin',(-84.8548278771908,-59.0746191263193,174.285485069079));
#46091=CARTESIAN_POINT('Origin',(-84.8548278771908,-59.0746191263193,174.285485069079));
#46092=CARTESIAN_POINT('Origin',(-99.6210548294771,-101.594714864612,178.585485069079));
#46093=CARTESIAN_POINT('',(-99.6210548299422,-101.594714864439,177.585485069079));
#46094=CARTESIAN_POINT('',(-99.6210548299422,-101.594714864439,174.385485069079));
#46095=CARTESIAN_POINT('',(-99.6210548294771,-101.594714864612,178.585485069079));
#46096=CARTESIAN_POINT('',(-99.1880632280731,-101.755948961215,174.385485069079));
#46097=CARTESIAN_POINT('',(-98.2153504257721,-102.118160305326,174.385485069079));
#46098=CARTESIAN_POINT('',(-99.1880632280731,-101.755948961215,177.585485069079));
#46099=CARTESIAN_POINT('',(-99.1880632280731,-101.755948961215,178.585485069079));
#46100=CARTESIAN_POINT('',(-99.6210548294771,-101.594714864612,177.585485069079));
#46101=CARTESIAN_POINT('Ctrl Pts',(-97.8838106736817,-101.114486609555,
174.371590892235));
#46102=CARTESIAN_POINT('Ctrl Pts',(-97.8838106736817,-101.114486609555,
173.188263904448));
#46103=CARTESIAN_POINT('Ctrl Pts',(-96.3541371085078,-96.1722845480714,
174.371590892235));
#46104=CARTESIAN_POINT('Ctrl Pts',(-96.3541371085078,-96.1722845480714,
173.188263904448));
#46105=CARTESIAN_POINT('Ctrl Pts',(-91.1365269123698,-76.1991465747503,
174.371590892235));
#46106=CARTESIAN_POINT('Ctrl Pts',(-91.1365269123698,-76.1991465747503,
173.188263904448));
#46107=CARTESIAN_POINT('Ctrl Pts',(-87.1439910232441,-64.4286763559758,
174.371590892235));
#46108=CARTESIAN_POINT('Ctrl Pts',(-87.1439910232441,-64.4286763559758,
173.188263904448));
#46109=CARTESIAN_POINT('Ctrl Pts',(-83.9950826197058,-63.9298573380069,
174.371590892235));
#46110=CARTESIAN_POINT('Ctrl Pts',(-83.9950826197058,-63.9298573380069,
173.188263904448));
#46111=CARTESIAN_POINT('Ctrl Pts',(-81.9013008568494,-58.3070397231869,
174.371590892235));
#46112=CARTESIAN_POINT('Ctrl Pts',(-81.9013008568494,-58.3070397231869,
173.188263904448));
#46113=CARTESIAN_POINT('',(-94.2301013700656,-88.1262479603296,174.285485110655));
#46114=CARTESIAN_POINT('',(-81.9013008568494,-58.3070397231869,174.285485069079));
#46115=CARTESIAN_POINT('Ctrl Pts',(-94.2301013700775,-88.1262479603088,
174.285485069079));
#46116=CARTESIAN_POINT('Ctrl Pts',(-92.4302378087403,-81.6315356194262,
174.285485069079));
#46117=CARTESIAN_POINT('Ctrl Pts',(-89.7937145858027,-72.240376274824,174.285485069079));
#46118=CARTESIAN_POINT('Ctrl Pts',(-87.1439910232441,-64.4286763559758,
174.285485069079));
#46119=CARTESIAN_POINT('Ctrl Pts',(-83.9950826197058,-63.9298573380069,
174.285485069079));
#46120=CARTESIAN_POINT('Ctrl Pts',(-81.9013008568494,-58.3070397231869,
174.285485069079));
#46121=CARTESIAN_POINT('',(-97.8838106717876,-101.114486603435,174.36571584827));
#46122=CARTESIAN_POINT('Ctrl Pts',(-94.2301013700819,-88.1262479603247,
174.285485152574));
#46123=CARTESIAN_POINT('Ctrl Pts',(-94.8572392714732,-90.3892418644711,
174.285505819717));
#46124=CARTESIAN_POINT('Ctrl Pts',(-95.4293953813936,-92.4665577589316,
174.289138567121));
#46125=CARTESIAN_POINT('Ctrl Pts',(-96.9354756174802,-97.8900543030279,
174.323115739585));
#46126=CARTESIAN_POINT('Ctrl Pts',(-97.5030442713843,-99.8842734829934,
174.356479113651));
#46127=CARTESIAN_POINT('Ctrl Pts',(-97.8838106717875,-101.114486603435,
174.36571584829));
#46128=CARTESIAN_POINT('',(-97.8838106723181,-101.11448660515,173.385485069079));
#46129=CARTESIAN_POINT('',(-97.8838106722024,-101.114486604776,174.285485069079));
#46130=CARTESIAN_POINT('',(-81.9013008568494,-58.3070397231869,173.385485069079));
#46131=CARTESIAN_POINT('Ctrl Pts',(-97.8838106722024,-101.114486604776,
173.385485069079));
#46132=CARTESIAN_POINT('Ctrl Pts',(-96.3541371055762,-96.1722845368492,
173.385485069079));
#46133=CARTESIAN_POINT('Ctrl Pts',(-91.1365269114412,-76.1991465720129,
173.385485069079));
#46134=CARTESIAN_POINT('Ctrl Pts',(-87.1439910232441,-64.4286763559758,
173.385485069079));
#46135=CARTESIAN_POINT('Ctrl Pts',(-83.9950826197058,-63.9298573380069,
173.385485069079));
#46136=CARTESIAN_POINT('Ctrl Pts',(-81.9013008568494,-58.3070397231869,
173.385485069079));
#46137=CARTESIAN_POINT('',(-81.9013008568494,-58.3070397231869,178.585485069079));
#46138=CARTESIAN_POINT('Origin',(-48.2819354919502,-57.24716229829,178.585485069079));
#46139=CARTESIAN_POINT('',(-80.6956086449654,-48.2616817644572,174.285485069079));
#46140=CARTESIAN_POINT('Origin',(-48.2819354919502,-57.24716229829,174.285485069079));
#46141=CARTESIAN_POINT('Origin',(-48.2819354919502,-57.24716229829,173.385485069079));
#46142=CARTESIAN_POINT('Ctrl Pts',(-77.0748911463595,-39.8589256890876,
174.590829198952));
#46143=CARTESIAN_POINT('Ctrl Pts',(-77.1258588534607,-39.9433224547489,
174.592143873877));
#46144=CARTESIAN_POINT('Ctrl Pts',(-77.1764462985522,-40.0279274916938,
174.593076422781));
#46145=CARTESIAN_POINT('Ctrl Pts',(-77.3118277495375,-40.2566253387939,
174.59465858183));
#46146=CARTESIAN_POINT('Ctrl Pts',(-77.3957878287932,-40.400899198962,174.594658945545));
#46147=CARTESIAN_POINT('Ctrl Pts',(-77.6960535448169,-40.9258180381849,
174.591863571298));
#46148=CARTESIAN_POINT('Ctrl Pts',(-77.9051062567381,-41.3082355654289,
174.584711888553));
#46149=CARTESIAN_POINT('Ctrl Pts',(-78.474706173954,-42.4011423337224,174.550066413528));
#46150=CARTESIAN_POINT('Ctrl Pts',(-78.8133875775858,-43.1109905067965,
174.512103266793));
#46151=CARTESIAN_POINT('Ctrl Pts',(-79.7866388893984,-45.3484841750064,
174.382338566305));
#46152=CARTESIAN_POINT('Ctrl Pts',(-80.3006668857753,-46.836993007004,174.28548333118));
#46153=CARTESIAN_POINT('Ctrl Pts',(-80.6956086449654,-48.261681764457,174.285485069103));
#46154=CARTESIAN_POINT('Origin',(-93.2994946198038,-77.3496518591637,178.585485069079));
#46155=CARTESIAN_POINT('',(-98.376517057274,-100.991065637145,178.585485066968));
#46156=CARTESIAN_POINT('',(-97.9019633317937,-101.167776319221,178.585485069079));
#46157=CARTESIAN_POINT('',(-101.649120271255,-99.7724387145074,178.585485069079));
#46158=CARTESIAN_POINT('',(-97.883810672318,-101.114486605149,178.585485069079));
#46159=CARTESIAN_POINT('Origin',(-98.8390996009304,-100.818812692078,178.585485069079));
#46160=CARTESIAN_POINT('',(-81.9013008568494,-58.3070397231869,178.585485069079));
#46161=CARTESIAN_POINT('Ctrl Pts',(-97.8838106722022,-101.114486604775,
178.585485069079));
#46162=CARTESIAN_POINT('Ctrl Pts',(-96.3541371055757,-96.1722845368475,
178.585485069079));
#46163=CARTESIAN_POINT('Ctrl Pts',(-91.1365269114411,-76.1991465720125,
178.585485069079));
#46164=CARTESIAN_POINT('Ctrl Pts',(-87.1439910232441,-64.4286763559758,
178.585485069079));
#46165=CARTESIAN_POINT('Ctrl Pts',(-83.9950826197058,-63.9298573380069,
178.585485069079));
#46166=CARTESIAN_POINT('Ctrl Pts',(-81.9013008568494,-58.3070397231869,
178.585485069079));
#46167=CARTESIAN_POINT('Origin',(-48.2819354919502,-57.24716229829,178.585485069079));
#46168=CARTESIAN_POINT('Ctrl Pts',(-77.4650015118695,-40.1676234768323,
178.585484783646));
#46169=CARTESIAN_POINT('Ctrl Pts',(-77.6905814020153,-40.555127005694,178.58548463742));
#46170=CARTESIAN_POINT('Ctrl Pts',(-77.9138848638019,-40.9434090043415,
178.585484508233));
#46171=CARTESIAN_POINT('Ctrl Pts',(-78.1332843656806,-41.3333760529069,
178.585484451998));
#46172=CARTESIAN_POINT('Ctrl Pts',(-78.4717618076451,-41.9349956915966,
178.585484365242));
#46173=CARTESIAN_POINT('Ctrl Pts',(-78.8029288442396,-42.5395302271617,
178.585484447149));
#46174=CARTESIAN_POINT('Ctrl Pts',(-79.1274796035695,-43.1466863215047,
178.585484576633));
#46175=CARTESIAN_POINT('Ctrl Pts',(-79.6250115124666,-44.07744837315,178.585484775131));
#46176=CARTESIAN_POINT('Ctrl Pts',(-80.1070311508828,-45.0143523211482,
178.585484994787));
#46177=CARTESIAN_POINT('Ctrl Pts',(-80.5756237742355,-45.9565750778124,
178.585485043419));
#46178=CARTESIAN_POINT('Ctrl Pts',(-80.719647585736,-46.2461709995885,178.585485058367));
#46179=CARTESIAN_POINT('Ctrl Pts',(-80.8624028290514,-46.5362697111046,
178.585485063812));
#46180=CARTESIAN_POINT('Ctrl Pts',(-81.0039496069982,-46.8268481729705,
178.58548506622));
#46181=CARTESIAN_POINT('Ctrl Pts',(-81.0837898722371,-46.9907506072371,
178.585485067579));
#46182=CARTESIAN_POINT('Ctrl Pts',(-81.1632479651378,-47.1548045771697,
178.585485068005));
#46183=CARTESIAN_POINT('Ctrl Pts',(-81.2423319510288,-47.3190072870547,
178.585485068133));
#46184=CARTESIAN_POINT('Ctrl Pts',(-81.8218342303691,-48.5222324859381,
178.585485069074));
#46185=CARTESIAN_POINT('Ctrl Pts',(-82.38085463941,-49.7335938646736,178.585485068901));
#46186=CARTESIAN_POINT('Ctrl Pts',(-82.9219084178718,-50.9520888272408,
178.58548506889));
#46187=CARTESIAN_POINT('Ctrl Pts',(-83.4244472543089,-52.0838451610268,
178.585485068881));
#46188=CARTESIAN_POINT('Ctrl Pts',(-83.9114855009559,-53.2217559573636,
178.585485068821));
#46189=CARTESIAN_POINT('Ctrl Pts',(-84.3850017277789,-54.3650338933268,
178.585485068922));
#46190=CARTESIAN_POINT('Ctrl Pts',(-84.4273715190481,-54.467333338975,178.585485068931));
#46191=CARTESIAN_POINT('Ctrl Pts',(-84.469632549005,-54.5696759937385,178.585485068941));
#46192=CARTESIAN_POINT('Ctrl Pts',(-84.5117857638681,-54.6720615186019,
178.585485068951));
#46193=CARTESIAN_POINT('Ctrl Pts',(-85.1131994842138,-56.1328293299712,
178.585485069102));
#46194=CARTESIAN_POINT('Ctrl Pts',(-85.6926892826506,-57.6023030610518,
178.585485069069));
#46195=CARTESIAN_POINT('Ctrl Pts',(-86.2529554615349,-59.0794092453283,
178.585485069072));
#46196=CARTESIAN_POINT('Ctrl Pts',(-86.6328377473246,-60.0809447561002,
178.585485069073));
#46197=CARTESIAN_POINT('Ctrl Pts',(-87.0038811370241,-61.0859896879636,
178.585485069073));
#46198=CARTESIAN_POINT('Ctrl Pts',(-87.3669151039208,-62.0942150904523,
178.585485069076));
#46199=CARTESIAN_POINT('Ctrl Pts',(-87.3769344349696,-62.1220409827942,
178.585485069076));
#46200=CARTESIAN_POINT('Ctrl Pts',(-87.3869476469901,-62.1498693064267,
178.585485069076));
#46201=CARTESIAN_POINT('Ctrl Pts',(-87.3969547526199,-62.1777000567301,
178.585485069076));
#46202=CARTESIAN_POINT('Ctrl Pts',(-88.0123319305732,-63.8891248398365,
178.585485069081));
#46203=CARTESIAN_POINT('Ctrl Pts',(-88.6046242589736,-65.6097164187148,
178.585485069081));
#46204=CARTESIAN_POINT('Ctrl Pts',(-89.1767249350884,-67.3383248097952,
178.585485069077));
#46205=CARTESIAN_POINT('Ctrl Pts',(-89.4481762250666,-68.1585178233966,
178.585485069076));
#46206=CARTESIAN_POINT('Ctrl Pts',(-89.7150809981247,-68.9805160269103,
178.585485069073));
#46207=CARTESIAN_POINT('Ctrl Pts',(-89.9777446627557,-69.8041983278515,
178.585485069061));
#46208=CARTESIAN_POINT('Ctrl Pts',(-89.9958921332768,-69.861106656973,178.58548506906));
#46209=CARTESIAN_POINT('Ctrl Pts',(-90.0140193906421,-69.91802307165,178.585485069059));
#46210=CARTESIAN_POINT('Ctrl Pts',(-90.0321265334954,-69.974947529394,178.585485069058));
#46211=CARTESIAN_POINT('Ctrl Pts',(-90.6556985380883,-71.9353064061813,
178.585485069019));
#46212=CARTESIAN_POINT('Ctrl Pts',(-91.2553870982626,-73.9057023814814,
178.585485068557));
#46213=CARTESIAN_POINT('Ctrl Pts',(-91.8342083922678,-75.8835284381501,
178.585485066831));
#46214=CARTESIAN_POINT('Ctrl Pts',(-92.4366613560735,-77.9421036531137,
178.585485065034));
#46215=CARTESIAN_POINT('Ctrl Pts',(-93.0165082496544,-80.0087281231012,
178.585485062237));
#46216=CARTESIAN_POINT('Ctrl Pts',(-93.5771032551113,-82.0804951687553,
178.585485063212));
#46217=CARTESIAN_POINT('Ctrl Pts',(-93.8691776689443,-83.1599021195265,
178.585485063719));
#46218=CARTESIAN_POINT('Ctrl Pts',(-94.1560254278893,-84.2407055417337,
178.585485065367));
#46219=CARTESIAN_POINT('Ctrl Pts',(-94.4381163838179,-85.3224975248452,
178.585485067051));
#46220=CARTESIAN_POINT('Ctrl Pts',(-94.5030528267729,-85.5715226067351,
178.585485067439));
#46221=CARTESIAN_POINT('Ctrl Pts',(-94.5677452759793,-85.8206032934907,
178.585485067419));
#46222=CARTESIAN_POINT('Ctrl Pts',(-94.6321980467042,-86.06973522053,178.585485067102));
#46223=CARTESIAN_POINT('Ctrl Pts',(-95.1418708908417,-88.039794480843,178.585485064593));
#46224=CARTESIAN_POINT('Ctrl Pts',(-95.6360250446987,-90.0141207468549,
178.585484976939));
#46225=CARTESIAN_POINT('Ctrl Pts',(-96.1219981705027,-91.9904905111795,
178.5854850137));
#46226=CARTESIAN_POINT('Ctrl Pts',(-96.2175637821243,-92.3791395439954,
178.585485020929));
#46227=CARTESIAN_POINT('Ctrl Pts',(-96.3128128668425,-92.7678675558309,
178.58548503405));
#46228=CARTESIAN_POINT('Ctrl Pts',(-96.4078010227875,-93.1566576401014,
178.585485047111));
#46229=CARTESIAN_POINT('Ctrl Pts',(-96.49385330348,-93.5088728518749,178.585485058943));
#46230=CARTESIAN_POINT('Ctrl Pts',(-96.5797668758499,-93.8611155073599,
178.585485057239));
#46231=CARTESIAN_POINT('Ctrl Pts',(-96.6655567819583,-94.2133925591645,
178.585485051882));
#46232=CARTESIAN_POINT('Ctrl Pts',(-96.8983471324597,-95.1692940408562,
178.585485037346));
#46233=CARTESIAN_POINT('Ctrl Pts',(-97.1298683277641,-96.1255675264222,
178.585484955934));
#46234=CARTESIAN_POINT('Ctrl Pts',(-97.3642924294251,-97.0810624897178,
178.585485025112));
#46235=CARTESIAN_POINT('Ctrl Pts',(-97.4633229695275,-97.4847035044845,
178.585485054336));
#46236=CARTESIAN_POINT('Ctrl Pts',(-97.5629746719815,-97.8881695057605,
178.585485062002));
#46237=CARTESIAN_POINT('Ctrl Pts',(-97.6636749002389,-98.2913808726464,
178.585485062489));
#46238=CARTESIAN_POINT('Ctrl Pts',(-97.7260872514047,-98.5412846698832,
178.585485062791));
#46239=CARTESIAN_POINT('Ctrl Pts',(-97.7888472641501,-98.7911089883279,
178.585485061828));
#46240=CARTESIAN_POINT('Ctrl Pts',(-97.8524422630192,-99.0407060185016,
178.585485047837));
#46241=CARTESIAN_POINT('Ctrl Pts',(-97.9614492780947,-99.4685356861605,
178.585485023857));
#46242=CARTESIAN_POINT('Ctrl Pts',(-98.072667959701,-99.8957209843174,178.585485018479));
#46243=CARTESIAN_POINT('Ctrl Pts',(-98.1886188504326,-100.321776749252,
178.585485035129));
#46244=CARTESIAN_POINT('Ctrl Pts',(-98.2494587013773,-100.545329747157,
178.585485043865));
#46245=CARTESIAN_POINT('Ctrl Pts',(-98.3115349193939,-100.768593902497,
178.585485055673));
#46246=CARTESIAN_POINT('Ctrl Pts',(-98.3765170572738,-100.991065637145,
178.585485062744));
#46247=CARTESIAN_POINT('Origin',(-93.2994946198038,-77.3496518591637,173.385485069079));
#46248=CARTESIAN_POINT('',(-97.9019633317937,-101.167776319221,173.385485069079));
#46249=CARTESIAN_POINT('Origin',(-98.8390996009304,-100.818812692078,173.385485069079));
#46250=CARTESIAN_POINT('',(-98.376517057274,-100.991065637145,173.385485071191));
#46251=CARTESIAN_POINT('',(-99.2720912023343,-100.657578595475,173.385485069079));
#46252=CARTESIAN_POINT('Ctrl Pts',(-98.3765170572737,-100.991065637145,
173.385485075415));
#46253=CARTESIAN_POINT('Ctrl Pts',(-98.311534919394,-100.768593902497,173.385485082486));
#46254=CARTESIAN_POINT('Ctrl Pts',(-98.2494587013798,-100.545329747159,
173.385485094294));
#46255=CARTESIAN_POINT('Ctrl Pts',(-98.1886188504344,-100.321776749251,
173.38548510303));
#46256=CARTESIAN_POINT('Ctrl Pts',(-98.0726679597014,-99.8957209843114,
173.38548511968));
#46257=CARTESIAN_POINT('Ctrl Pts',(-97.9614492780947,-99.4685356861606,
173.385485114302));
#46258=CARTESIAN_POINT('Ctrl Pts',(-97.8524422630192,-99.0407060185016,
173.385485090321));
#46259=CARTESIAN_POINT('Ctrl Pts',(-97.7888472641501,-98.7911089883279,
173.385485076331));
#46260=CARTESIAN_POINT('Ctrl Pts',(-97.7260872514046,-98.5412846698841,
173.385485075368));
#46261=CARTESIAN_POINT('Ctrl Pts',(-97.6636749002385,-98.2913808726465,
173.38548507567));
#46262=CARTESIAN_POINT('Ctrl Pts',(-97.5629746719806,-97.8881695057594,
173.385485076157));
#46263=CARTESIAN_POINT('Ctrl Pts',(-97.4633229695275,-97.4847035044845,
173.385485083822));
#46264=CARTESIAN_POINT('Ctrl Pts',(-97.3642924294252,-97.0810624897179,
173.385485113046));
#46265=CARTESIAN_POINT('Ctrl Pts',(-97.129868327764,-96.1255675264219,173.385485182225));
#46266=CARTESIAN_POINT('Ctrl Pts',(-96.8983471324719,-95.1692940408548,
173.385485100813));
#46267=CARTESIAN_POINT('Ctrl Pts',(-96.6655567819617,-94.2133925591637,
173.385485086277));
#46268=CARTESIAN_POINT('Ctrl Pts',(-96.5797668758502,-93.8611155073597,
173.38548508092));
#46269=CARTESIAN_POINT('Ctrl Pts',(-96.4938533034791,-93.5088728518748,
173.385485079216));
#46270=CARTESIAN_POINT('Ctrl Pts',(-96.4078010227867,-93.1566576401016,
173.385485091048));
#46271=CARTESIAN_POINT('Ctrl Pts',(-95.9247643984986,-91.1795706233595,
173.385485157466));
#46272=CARTESIAN_POINT('Ctrl Pts',(-95.4349837366555,-89.2040886563437,
173.385485090674));
#46273=CARTESIAN_POINT('Ctrl Pts',(-94.9311314986831,-87.2324375352915,
173.385485075759));
#46274=CARTESIAN_POINT('Ctrl Pts',(-94.8320499884367,-86.844716382084,173.385485072826));
#46275=CARTESIAN_POINT('Ctrl Pts',(-94.7324241658693,-86.4571433323539,
173.38548507155));
#46276=CARTESIAN_POINT('Ctrl Pts',(-94.6321980466999,-86.0697352205311,
173.385485071057));
#46277=CARTESIAN_POINT('Ctrl Pts',(-94.567745275975,-85.8206032934928,173.38548507074));
#46278=CARTESIAN_POINT('Ctrl Pts',(-94.5030528267687,-85.5715226067371,
173.38548507072));
#46279=CARTESIAN_POINT('Ctrl Pts',(-94.4381163838136,-85.3224975248463,
173.385485071108));
#46280=CARTESIAN_POINT('Ctrl Pts',(-93.8936936520863,-83.2346881348964,
173.385485074359));
#46281=CARTESIAN_POINT('Ctrl Pts',(-93.3315556794994,-81.1505590794656,
173.385485075867));
#46282=CARTESIAN_POINT('Ctrl Pts',(-92.7483148961997,-79.0730496714838,
173.385485074267));
#46283=CARTESIAN_POINT('Ctrl Pts',(-92.1887794724172,-77.0799789873133,
173.385485072732));
#46284=CARTESIAN_POINT('Ctrl Pts',(-91.6098219083077,-75.0930006983604,
173.385485070307));
#46285=CARTESIAN_POINT('Ctrl Pts',(-91.0084120392233,-73.1147375455329,
173.385485069579));
#46286=CARTESIAN_POINT('Ctrl Pts',(-90.6894518180546,-72.0655574685308,
173.385485069193));
#46287=CARTESIAN_POINT('Ctrl Pts',(-90.3641756334622,-71.0188292236311,
173.385485069122));
#46288=CARTESIAN_POINT('Ctrl Pts',(-90.0321265335055,-69.9749475293908,
173.385485069101));
#46289=CARTESIAN_POINT('Ctrl Pts',(-90.0140193906523,-69.9180230716466,
173.3854850691));
#46290=CARTESIAN_POINT('Ctrl Pts',(-89.9958921332871,-69.8611066569696,
173.385485069099));
#46291=CARTESIAN_POINT('Ctrl Pts',(-89.9777446627662,-69.8041983278482,
173.385485069098));
#46292=CARTESIAN_POINT('Ctrl Pts',(-89.4241644259319,-68.068235937028,173.385485069073));
#46293=CARTESIAN_POINT('Ctrl Pts',(-88.8517488584057,-66.3397526068269,
173.385485069079));
#46294=CARTESIAN_POINT('Ctrl Pts',(-88.2576270599827,-64.6198876182801,
173.38548506908));
#46295=CARTESIAN_POINT('Ctrl Pts',(-87.9757272049345,-63.8038433454379,
173.38548506908));
#46296=CARTESIAN_POINT('Ctrl Pts',(-87.6889399119433,-62.9897396575733,
173.385485069081));
#46297=CARTESIAN_POINT('Ctrl Pts',(-87.3969547526246,-62.1777000567284,
173.385485069083));
#46298=CARTESIAN_POINT('Ctrl Pts',(-87.3869476469948,-62.1498693064251,
173.385485069083));
#46299=CARTESIAN_POINT('Ctrl Pts',(-87.3769344349743,-62.1220409827925,
173.385485069083));
#46300=CARTESIAN_POINT('Ctrl Pts',(-87.3669151039254,-62.0942150904507,
173.385485069083));
#46301=CARTESIAN_POINT('Ctrl Pts',(-86.8314975075075,-60.6072423251777,
173.385485069087));
#46302=CARTESIAN_POINT('Ctrl Pts',(-86.278660184972,-59.1271866439569,173.385485069082));
#46303=CARTESIAN_POINT('Ctrl Pts',(-85.7057349163769,-57.6551066868731,
173.385485069093));
#46304=CARTESIAN_POINT('Ctrl Pts',(-85.317269307623,-56.6569792381303,173.3854850691));
#46305=CARTESIAN_POINT('Ctrl Pts',(-84.9195676645059,-55.6625189265031,
173.385485069105));
#46306=CARTESIAN_POINT('Ctrl Pts',(-84.5117857638601,-54.6720615186052,
173.385485069208));
#46307=CARTESIAN_POINT('Ctrl Pts',(-84.4696325489975,-54.569675993742,173.385485069218));
#46308=CARTESIAN_POINT('Ctrl Pts',(-84.4273715190409,-54.4673333389783,
173.385485069228));
#46309=CARTESIAN_POINT('Ctrl Pts',(-84.3850017277721,-54.3650338933295,
173.385485069237));
#46310=CARTESIAN_POINT('Ctrl Pts',(-83.8751948703674,-53.1341342986271,
173.385485069345));
#46311=CARTESIAN_POINT('Ctrl Pts',(-83.3497144088603,-51.9094558257061,
173.385485069266));
#46312=CARTESIAN_POINT('Ctrl Pts',(-82.8060894939277,-50.6919817529054,
173.385485069267));
#46313=CARTESIAN_POINT('Ctrl Pts',(-82.3011625525949,-49.5611736481895,
173.385485069268));
#46314=CARTESIAN_POINT('Ctrl Pts',(-81.7805823269495,-48.4365808302589,
173.385485069152));
#46315=CARTESIAN_POINT('Ctrl Pts',(-81.2423319510283,-47.3190072870549,
173.385485070025));
#46316=CARTESIAN_POINT('Ctrl Pts',(-81.1632479651373,-47.15480457717,173.385485070154));
#46317=CARTESIAN_POINT('Ctrl Pts',(-81.0837898722368,-46.9907506072374,
173.38548507058));
#46318=CARTESIAN_POINT('Ctrl Pts',(-81.003949606998,-46.8268481729707,173.385485071939));
#46319=CARTESIAN_POINT('Ctrl Pts',(-80.5434162035343,-45.8814286448278,
173.385485079774));
#46320=CARTESIAN_POINT('Ctrl Pts',(-80.0700920299859,-44.9410842957925,
173.385485162657));
#46321=CARTESIAN_POINT('Ctrl Pts',(-79.5818989661386,-44.0066238667974,
173.385485368229));
#46322=CARTESIAN_POINT('Ctrl Pts',(-79.4318508819061,-43.7194137289541,
173.385485431413));
#46323=CARTESIAN_POINT('Ctrl Pts',(-79.2803980192546,-43.432759748701,173.385485500516));
#46324=CARTESIAN_POINT('Ctrl Pts',(-79.1274796035642,-43.1466863215074,
173.385485561525));
#46325=CARTESIAN_POINT('Ctrl Pts',(-78.8029288442143,-42.5395302271525,
173.38548569101));
#46326=CARTESIAN_POINT('Ctrl Pts',(-78.4717618076259,-41.9349956915895,
173.385485772917));
#46327=CARTESIAN_POINT('Ctrl Pts',(-78.1332843656745,-41.3333760529103,
173.385485686161));
#46328=CARTESIAN_POINT('Ctrl Pts',(-77.9138848638038,-40.9434090043507,
173.385485629926));
#46329=CARTESIAN_POINT('Ctrl Pts',(-77.6905814020163,-40.5551270056959,
173.385485500739));
#46330=CARTESIAN_POINT('Ctrl Pts',(-77.4650015118694,-40.1676234768323,
173.385485354513));
#46331=CARTESIAN_POINT('Ctrl Pts',(-78.158666194104,-39.3728065519909,177.585485069079));
#46332=CARTESIAN_POINT('Ctrl Pts',(-78.158666194104,-39.3728065519909,173.745485069079));
#46333=CARTESIAN_POINT('Ctrl Pts',(-91.6625086178529,-62.3675309666402,
177.585485069079));
#46334=CARTESIAN_POINT('Ctrl Pts',(-91.6625086178529,-62.3675309666402,
173.745485069079));
#46335=CARTESIAN_POINT('Ctrl Pts',(-97.8762366937634,-96.9090335189287,
177.585485069079));
#46336=CARTESIAN_POINT('Ctrl Pts',(-97.8762366937634,-96.9090335189287,
173.745485069079));
#46337=CARTESIAN_POINT('Ctrl Pts',(-99.6210548294771,-101.594714864612,
177.585485069079));
#46338=CARTESIAN_POINT('Ctrl Pts',(-99.6210548294771,-101.594714864612,
173.745485069079));
#46339=CARTESIAN_POINT('Ctrl Pts',(-78.158666194104,-39.372806551991,174.385485069079));
#46340=CARTESIAN_POINT('Ctrl Pts',(-79.5634562342768,-41.7649227231192,
174.385485069079));
#46341=CARTESIAN_POINT('Ctrl Pts',(-80.8467635159852,-44.2054723433059,
174.385485069079));
#46342=CARTESIAN_POINT('Ctrl Pts',(-83.2418725976757,-49.1549483814856,
174.385485069079));
#46343=CARTESIAN_POINT('Ctrl Pts',(-84.3529474705451,-51.6641646149859,
174.385485069079));
#46344=CARTESIAN_POINT('Ctrl Pts',(-86.4442463955118,-56.7347654443307,
174.385485069079));
#46345=CARTESIAN_POINT('Ctrl Pts',(-87.4241628164095,-59.2962726883618,
174.385485069079));
#46346=CARTESIAN_POINT('Ctrl Pts',(-89.2799424409765,-64.4607717151331,
174.385485069079));
#46347=CARTESIAN_POINT('Ctrl Pts',(-90.1556460538296,-67.0638271244634,
174.385485069079));
#46348=CARTESIAN_POINT('Ctrl Pts',(-92.6553603269606,-74.9237845522913,
174.385485069079));
#46349=CARTESIAN_POINT('Ctrl Pts',(-94.1520335629162,-80.2352141170513,
174.385485069079));
#46350=CARTESIAN_POINT('Ctrl Pts',(-96.2277705472134,-88.2383598976106,
174.385485069079));
#46351=CARTESIAN_POINT('Ctrl Pts',(-96.8905903551983,-90.913701399124,174.385485069079));
#46352=CARTESIAN_POINT('Ctrl Pts',(-97.8694497883241,-94.9305941684308,
174.385485069079));
#46353=CARTESIAN_POINT('Ctrl Pts',(-98.1926873948002,-96.27033732199,174.385485069079));
#46354=CARTESIAN_POINT('Ctrl Pts',(-98.6897521666471,-98.2768331740868,
174.385485069079));
#46355=CARTESIAN_POINT('Ctrl Pts',(-98.8572817108174,-98.9451947300226,
174.385485069079));
#46356=CARTESIAN_POINT('Ctrl Pts',(-99.1212462758668,-99.9445001871973,
174.385485069079));
#46357=CARTESIAN_POINT('Ctrl Pts',(-99.2113105712096,-100.277071621847,
174.385485069079));
#46358=CARTESIAN_POINT('Ctrl Pts',(-99.4021032609997,-100.939490126788,
174.385485069079));
#46359=CARTESIAN_POINT('Ctrl Pts',(-99.500148440254,-101.270022679816,174.385485069079));
#46360=CARTESIAN_POINT('Ctrl Pts',(-99.6210548294771,-101.594714864612,
174.385485069079));
#46361=CARTESIAN_POINT('Ctrl Pts',(-99.6210548294771,-101.594714864612,
177.585485069079));
#46362=CARTESIAN_POINT('Ctrl Pts',(-99.5610285400747,-101.433515219282,
177.585485069079));
#46363=CARTESIAN_POINT('Ctrl Pts',(-99.5069208217296,-101.268946229191,
177.585485069079));
#46364=CARTESIAN_POINT('Ctrl Pts',(-99.4038032743778,-100.940304890532,
177.585485069079));
#46365=CARTESIAN_POINT('Ctrl Pts',(-99.3548261927294,-100.775311081876,
177.585485069079));
#46366=CARTESIAN_POINT('Ctrl Pts',(-99.2119254375992,-100.279278763247,
177.585485069079));
#46367=CARTESIAN_POINT('Ctrl Pts',(-99.1219766295885,-99.9472038638691,
177.585485069079));
#46368=CARTESIAN_POINT('Ctrl Pts',(-98.8583492039865,-98.9493576507077,
177.585485069079));
#46369=CARTESIAN_POINT('Ctrl Pts',(-98.691030413114,-98.2819281029329,177.585485069079));
#46370=CARTESIAN_POINT('Ctrl Pts',(-98.1946027213088,-96.2781979350422,
177.585485069079));
#46371=CARTESIAN_POINT('Ctrl Pts',(-97.8717928229948,-94.9402549399502,
177.585485069079));
#46372=CARTESIAN_POINT('Ctrl Pts',(-96.8942898157684,-90.9287916912753,
177.585485069079));
#46373=CARTESIAN_POINT('Ctrl Pts',(-96.2324745724884,-88.2571284325171,
177.585485069079));
#46374=CARTESIAN_POINT('Ctrl Pts',(-94.1600380638105,-80.2648202595016,
177.585485069079));
#46375=CARTESIAN_POINT('Ctrl Pts',(-92.6665566865773,-74.9615276259966,
177.585485069079));
#46376=CARTESIAN_POINT('Ctrl Pts',(-90.1657169570279,-67.0942364364973,
177.585485069079));
#46377=CARTESIAN_POINT('Ctrl Pts',(-89.289147208604,-64.4872953405147,177.585485069079));
#46378=CARTESIAN_POINT('Ctrl Pts',(-87.4300065178477,-59.3116351672732,
177.585485069079));
#46379=CARTESIAN_POINT('Ctrl Pts',(-86.4476068577322,-56.7428543288977,
177.585485069079));
#46380=CARTESIAN_POINT('Ctrl Pts',(-84.3486009704813,-51.6536849931039,
177.585485069079));
#46381=CARTESIAN_POINT('Ctrl Pts',(-83.2324817482337,-49.1343169853156,
177.585485069079));
#46382=CARTESIAN_POINT('Ctrl Pts',(-80.8356389933579,-44.1837194009194,
177.585485069079));
#46383=CARTESIAN_POINT('Ctrl Pts',(-79.554497878766,-41.7496681822473,177.585485069079));
#46384=CARTESIAN_POINT('Ctrl Pts',(-78.158666194104,-39.372806551991,177.585485069079));
#46385=CARTESIAN_POINT('Ctrl Pts',(-97.8838106736817,-101.114486609555,
178.585485069079));
#46386=CARTESIAN_POINT('Ctrl Pts',(-97.8838106736817,-101.114486609555,
177.402158081293));
#46387=CARTESIAN_POINT('Ctrl Pts',(-96.3541371085078,-96.1722845480715,
178.585485069079));
#46388=CARTESIAN_POINT('Ctrl Pts',(-96.3541371085078,-96.1722845480715,
177.402158081293));
#46389=CARTESIAN_POINT('Ctrl Pts',(-91.1365269123698,-76.1991465747503,
178.585485069079));
#46390=CARTESIAN_POINT('Ctrl Pts',(-91.1365269123698,-76.1991465747503,
177.402158081293));
#46391=CARTESIAN_POINT('Ctrl Pts',(-87.1439910232441,-64.4286763559758,
178.585485069079));
#46392=CARTESIAN_POINT('Ctrl Pts',(-87.1439910232441,-64.4286763559758,
177.402158081293));
#46393=CARTESIAN_POINT('Ctrl Pts',(-83.9950826197058,-63.9298573380069,
178.585485069079));
#46394=CARTESIAN_POINT('Ctrl Pts',(-83.9950826197058,-63.9298573380069,
177.402158081293));
#46395=CARTESIAN_POINT('Ctrl Pts',(-81.9013008568494,-58.3070397231869,
178.585485069079));
#46396=CARTESIAN_POINT('Ctrl Pts',(-81.9013008568494,-58.3070397231869,
177.402158081293));
#46397=CARTESIAN_POINT('',(-97.8838106717876,-101.114486603436,177.605254289888));
#46398=CARTESIAN_POINT('',(-97.8838106722024,-101.114486604776,178.585485069079));
#46399=CARTESIAN_POINT('',(-94.2301013700811,-88.1262479603857,177.685485027504));
#46400=CARTESIAN_POINT('Ctrl Pts',(-97.8838106717875,-101.114486603435,
177.605254289869));
#46401=CARTESIAN_POINT('Ctrl Pts',(-97.5030442961786,-99.8842735631011,
177.614491023905));
#46402=CARTESIAN_POINT('Ctrl Pts',(-96.9354756924371,-97.8900545660898,
177.647854393757));
#46403=CARTESIAN_POINT('Ctrl Pts',(-95.4293955181978,-92.466558256121,177.681831570023));
#46404=CARTESIAN_POINT('Ctrl Pts',(-94.8572393589048,-90.3892421799639,
177.685464318439));
#46405=CARTESIAN_POINT('Ctrl Pts',(-94.2301013700974,-88.1262479603808,
177.685484985585));
#46406=CARTESIAN_POINT('',(-81.9013008568494,-58.3070397231869,177.685485069079));
#46407=CARTESIAN_POINT('Ctrl Pts',(-94.230101370093,-88.1262479603649,177.685485069079));
#46408=CARTESIAN_POINT('Ctrl Pts',(-92.4302378087522,-81.6315356194686,
177.685485069079));
#46409=CARTESIAN_POINT('Ctrl Pts',(-89.7937145858072,-72.240376274837,177.685485069079));
#46410=CARTESIAN_POINT('Ctrl Pts',(-87.1439910232441,-64.4286763559758,
177.685485069079));
#46411=CARTESIAN_POINT('Ctrl Pts',(-83.9950826197058,-63.9298573380069,
177.685485069079));
#46412=CARTESIAN_POINT('Ctrl Pts',(-81.9013008568494,-58.3070397231869,
177.685485069079));
#46413=CARTESIAN_POINT('',(-81.9013008568494,-58.3070397231869,178.585485069079));
#46414=CARTESIAN_POINT('Origin',(-48.2819354919502,-57.24716229829,178.585485069079));
#46415=CARTESIAN_POINT('',(-80.6956086449674,-48.2616817644643,177.685485069079));
#46416=CARTESIAN_POINT('Origin',(-48.2819354919502,-57.24716229829,177.685485069079));
#46417=CARTESIAN_POINT('Ctrl Pts',(-80.6956086449673,-48.2616817644641,
177.685485069056));
#46418=CARTESIAN_POINT('Ctrl Pts',(-80.3006668909431,-46.8369930256451,
177.685486806981));
#46419=CARTESIAN_POINT('Ctrl Pts',(-79.7866389024401,-45.3484842121757,
177.588631574318));
#46420=CARTESIAN_POINT('Ctrl Pts',(-78.8133875980925,-43.1109905505337,
177.458866873764));
#46421=CARTESIAN_POINT('Ctrl Pts',(-78.4747061907265,-42.4011423672079,
177.420903726026));
#46422=CARTESIAN_POINT('Ctrl Pts',(-77.9051062662601,-41.3082355829664,
177.386258249981));
#46423=CARTESIAN_POINT('Ctrl Pts',(-77.6960535523287,-40.9258180515529,
177.379106567025));
#46424=CARTESIAN_POINT('Ctrl Pts',(-77.3957878325661,-40.4008992054676,
177.376311192626));
#46425=CARTESIAN_POINT('Ctrl Pts',(-77.3118277525961,-40.2566253440053,
177.376311556297));
#46426=CARTESIAN_POINT('Ctrl Pts',(-77.1764463001175,-40.0279274943117,
177.377893715319));
#46427=CARTESIAN_POINT('Ctrl Pts',(-77.1258588542569,-39.9433224560675,
177.378826264229));
#46428=CARTESIAN_POINT('Ctrl Pts',(-77.0748911463744,-39.8589256891122,
177.380140939181));
#46429=CARTESIAN_POINT('Origin',(-93.2994946198038,-77.3496518591637,177.685485069079));
#46430=CARTESIAN_POINT('Ctrl Pts',(-94.2301013700599,-88.1262479603733,
177.685484985585));
#46431=CARTESIAN_POINT('Ctrl Pts',(-93.7609037487217,-86.2787775829358,
177.685484911581));
#46432=CARTESIAN_POINT('Ctrl Pts',(-93.2798504860541,-84.4344939240166,
177.68548504784));
#46433=CARTESIAN_POINT('Ctrl Pts',(-92.7836854151622,-82.5942786034907,
177.685485064168));
#46434=CARTESIAN_POINT('Ctrl Pts',(-92.6359385547694,-82.0463036411146,
177.68548506903));
#46435=CARTESIAN_POINT('Ctrl Pts',(-92.4868514135393,-81.4986892569901,
177.685485068967));
#46436=CARTESIAN_POINT('Ctrl Pts',(-92.3363371949808,-80.9514582278748,
177.685485069002));
#46437=CARTESIAN_POINT('Ctrl Pts',(-92.3269664573115,-80.917388633205,177.685485069004));
#46438=CARTESIAN_POINT('Ctrl Pts',(-92.317590034494,-80.883320423089,177.685485069007));
#46439=CARTESIAN_POINT('Ctrl Pts',(-92.3082079016947,-80.849253605753,177.685485069009));
#46440=CARTESIAN_POINT('Ctrl Pts',(-91.7304217636379,-78.751294085718,177.685485069135));
#46441=CARTESIAN_POINT('Ctrl Pts',(-91.1316580244191,-76.6586040978249,
177.685485069079));
#46442=CARTESIAN_POINT('Ctrl Pts',(-90.5086916305028,-74.5750064731804,
177.685485069079));
#46443=CARTESIAN_POINT('Ctrl Pts',(-90.4336469891343,-74.324009247608,177.685485069079));
#46444=CARTESIAN_POINT('Ctrl Pts',(-90.3582510931399,-74.0731440131607,
177.685485069079));
#46445=CARTESIAN_POINT('Ctrl Pts',(-90.2824982722455,-73.8224174920625,
177.685485069079));
#46446=CARTESIAN_POINT('Ctrl Pts',(-89.917539583476,-72.6144780213029,177.685485069079));
#46447=CARTESIAN_POINT('Ctrl Pts',(-89.5441964515263,-71.409423930501,177.685485069079));
#46448=CARTESIAN_POINT('Ctrl Pts',(-89.1617955303327,-70.2079449176487,
177.685485069079));
#46449=CARTESIAN_POINT('Ctrl Pts',(-88.6527415452668,-68.6085301527561,
177.685485069079));
#46450=CARTESIAN_POINT('Ctrl Pts',(-88.1276036690571,-67.0148515066794,
177.685485069079));
#46451=CARTESIAN_POINT('Ctrl Pts',(-87.5839489126203,-65.4278719429401,
177.685485069079));
#46452=CARTESIAN_POINT('Ctrl Pts',(-87.0553314119355,-63.8847875484985,
177.685485069079));
#46453=CARTESIAN_POINT('Ctrl Pts',(-86.5092073119288,-62.34803672185,177.685485069079));
#46454=CARTESIAN_POINT('Ctrl Pts',(-85.9432952559966,-60.8185262246806,
177.685485069079));
#46455=CARTESIAN_POINT('Ctrl Pts',(-85.8157986536034,-60.4739366552068,
177.685485069079));
#46456=CARTESIAN_POINT('Ctrl Pts',(-85.6872974782193,-60.129714676371,177.685485069079));
#46457=CARTESIAN_POINT('Ctrl Pts',(-85.5577653075821,-59.7858708180288,
177.685485069079));
#46458=CARTESIAN_POINT('Ctrl Pts',(-84.9035795890701,-58.0758081979705,
177.685485069079));
#46459=CARTESIAN_POINT('Ctrl Pts',(-84.4380969044864,-56.8776880926409,
177.685485069079));
#46460=CARTESIAN_POINT('Ctrl Pts',(-83.9593907228013,-55.6843887421588,
177.685485069075));
#46461=CARTESIAN_POINT('Ctrl Pts',(-83.4654560220973,-54.4966313344464,
177.685485068972));
#46462=CARTESIAN_POINT('Ctrl Pts',(-82.9903344236191,-53.3541135130576,
177.685485068874));
#46463=CARTESIAN_POINT('Ctrl Pts',(-82.5011223788676,-52.2167234425755,
177.685485068703));
#46464=CARTESIAN_POINT('Ctrl Pts',(-81.9959927121058,-51.0851245641857,
177.685485068751));
#46465=CARTESIAN_POINT('Ctrl Pts',(-81.6680421620932,-50.3504449383769,
177.685485068781));
#46466=CARTESIAN_POINT('Ctrl Pts',(-81.3333812632274,-49.6182068120372,
177.685485068931));
#46467=CARTESIAN_POINT('Ctrl Pts',(-80.991499413137,-48.8885971288398,177.68548506903));
#46468=CARTESIAN_POINT('Ctrl Pts',(-80.8934759176747,-48.6794052941422,
177.685485069058));
#46469=CARTESIAN_POINT('Ctrl Pts',(-80.794854333503,-48.4704314543238,177.685485069079));
#46470=CARTESIAN_POINT('Ctrl Pts',(-80.6956167008178,-48.2616828347543,
177.685485069079));
#46471=CARTESIAN_POINT('Origin',(-93.2994946198038,-77.3496518591637,174.285485069079));
#46472=CARTESIAN_POINT('Ctrl Pts',(-80.695616700829,-48.261682834749,174.285485069079));
#46473=CARTESIAN_POINT('Ctrl Pts',(-80.7948543335137,-48.4704314543193,
174.285485069079));
#46474=CARTESIAN_POINT('Ctrl Pts',(-80.8934759176831,-48.6794052941381,
174.2854850691));
#46475=CARTESIAN_POINT('Ctrl Pts',(-80.9914994131414,-48.888597128836,174.285485069129));
#46476=CARTESIAN_POINT('Ctrl Pts',(-81.5156771503982,-50.007244265953,174.28548506928));
#46477=CARTESIAN_POINT('Ctrl Pts',(-82.0228825597661,-51.1320690378344,
174.285485069461));
#46478=CARTESIAN_POINT('Ctrl Pts',(-82.5149477029265,-52.2624018736989,
174.285485069392));
#46479=CARTESIAN_POINT('Ctrl Pts',(-83.0257505562677,-53.4357774842463,
174.28548506932));
#46480=CARTESIAN_POINT('Ctrl Pts',(-83.5202380124723,-54.615088703677,174.28548506915));
#46481=CARTESIAN_POINT('Ctrl Pts',(-84.0004086366806,-55.7996123684871,
174.285485069105));
#46482=CARTESIAN_POINT('Ctrl Pts',(-84.3071383529486,-56.556277997958,174.285485069076));
#46483=CARTESIAN_POINT('Ctrl Pts',(-84.6080249651107,-57.3150711201698,
174.285485069079));
#46484=CARTESIAN_POINT('Ctrl Pts',(-84.9035795890703,-58.0758081979706,
174.285485069079));
#46485=CARTESIAN_POINT('Ctrl Pts',(-85.5577653075812,-59.7858708180264,
174.285485069079));
#46486=CARTESIAN_POINT('Ctrl Pts',(-86.1320133072127,-61.3102152867964,
174.285485069079));
#46487=CARTESIAN_POINT('Ctrl Pts',(-86.6860022344115,-62.8419893984846,
174.285485069079));
#46488=CARTESIAN_POINT('Ctrl Pts',(-87.2220157058671,-64.3802846100018,
174.285485069079));
#46489=CARTESIAN_POINT('Ctrl Pts',(-87.772984453019,-65.9614996924093,174.285485069079));
#46490=CARTESIAN_POINT('Ctrl Pts',(-88.3049605725574,-67.5496048953572,
174.285485069079));
#46491=CARTESIAN_POINT('Ctrl Pts',(-88.8203747377026,-69.1436372841121,
174.285485069079));
#46492=CARTESIAN_POINT('Ctrl Pts',(-88.9349920760239,-69.4981167725554,
174.285485069079));
#46493=CARTESIAN_POINT('Ctrl Pts',(-89.0487902001326,-69.8528894638316,
174.285485069079));
#46494=CARTESIAN_POINT('Ctrl Pts',(-89.1617955303599,-70.207944917638,174.285485069079));
#46495=CARTESIAN_POINT('Ctrl Pts',(-89.5441964515462,-71.4094239304843,
174.285485069079));
#46496=CARTESIAN_POINT('Ctrl Pts',(-89.9175395834869,-72.6144780212793,
174.285485069079));
#46497=CARTESIAN_POINT('Ctrl Pts',(-90.2824982722559,-73.8224174920276,
174.285485069079));
#46498=CARTESIAN_POINT('Ctrl Pts',(-90.9113434606063,-75.9037679225675,
174.285485069079));
#46499=CARTESIAN_POINT('Ctrl Pts',(-91.5155952534419,-77.9946739428601,
174.285485069044));
#46500=CARTESIAN_POINT('Ctrl Pts',(-92.098482701032,-80.0913078783335,174.285485069115));
#46501=CARTESIAN_POINT('Ctrl Pts',(-92.1686992971666,-80.3438755033487,
174.285485069124));
#46502=CARTESIAN_POINT('Ctrl Pts',(-92.2386058266307,-80.5965262964667,
174.285485069135));
#46503=CARTESIAN_POINT('Ctrl Pts',(-92.308207901702,-80.8492536057496,174.28548506915));
#46504=CARTESIAN_POINT('Ctrl Pts',(-92.3175900344974,-80.8833204230718,
174.285485069152));
#46505=CARTESIAN_POINT('Ctrl Pts',(-92.326966457311,-80.9173886331741,174.285485069154));
#46506=CARTESIAN_POINT('Ctrl Pts',(-92.3363371949764,-80.95145822783,174.285485069157));
#46507=CARTESIAN_POINT('Ctrl Pts',(-92.8417956348715,-82.7891752547728,
174.285485069276));
#46508=CARTESIAN_POINT('Ctrl Pts',(-93.3311638475814,-84.6312179529252,
174.285485143859));
#46509=CARTESIAN_POINT('Ctrl Pts',(-93.8077114875544,-86.4767126138309,
174.285485171775));
#46510=CARTESIAN_POINT('Ctrl Pts',(-93.9496167188407,-87.0262596574556,
174.285485180087));
#46511=CARTESIAN_POINT('Ctrl Pts',(-94.0903848106434,-87.5761125951912,
174.28548517461));
#46512=CARTESIAN_POINT('Ctrl Pts',(-94.2301013700444,-88.1262479603172,
174.285485152574));
#46513=CARTESIAN_POINT('Ctrl Pts',(-77.3304501603129,-39.7397688129298,
177.705885069079));
#46514=CARTESIAN_POINT('Ctrl Pts',(-77.3304501603129,-39.7397688129298,
173.576925069079));
#46515=CARTESIAN_POINT('Ctrl Pts',(-77.4354809475772,-39.918618205007,177.705885069079));
#46516=CARTESIAN_POINT('Ctrl Pts',(-77.4354809475772,-39.918618205007,173.576925069079));
#46517=CARTESIAN_POINT('Ctrl Pts',(-77.5387174074033,-40.095017410943,177.705885069079));
#46518=CARTESIAN_POINT('Ctrl Pts',(-77.5387174074033,-40.095017410943,173.576925069079));
#46519=CARTESIAN_POINT('Ctrl Pts',(-77.7452188224523,-40.4514138749057,
177.705885069079));
#46520=CARTESIAN_POINT('Ctrl Pts',(-77.7452188224523,-40.4514138749057,
173.576925069079));
#46521=CARTESIAN_POINT('Ctrl Pts',(-78.0537048438588,-40.988104564515,177.705885069079));
#46522=CARTESIAN_POINT('Ctrl Pts',(-78.0537048438588,-40.988104564515,173.576925069079));
#46523=CARTESIAN_POINT('Ctrl Pts',(-78.7646561081799,-42.2546401779696,
177.705885069079));
#46524=CARTESIAN_POINT('Ctrl Pts',(-78.7646561081799,-42.2546401779696,
173.576925069079));
#46525=CARTESIAN_POINT('Ctrl Pts',(-79.358919965841,-43.3632613763041,177.705885069079));
#46526=CARTESIAN_POINT('Ctrl Pts',(-79.358919965841,-43.3632613763041,173.576925069079));
#46527=CARTESIAN_POINT('Ctrl Pts',(-80.5274284163852,-45.6074041562991,
177.705885069079));
#46528=CARTESIAN_POINT('Ctrl Pts',(-80.5274284163852,-45.6074041562991,
173.576925069079));
#46529=CARTESIAN_POINT('Ctrl Pts',(-81.2797370189181,-47.139365595286,177.705885069079));
#46530=CARTESIAN_POINT('Ctrl Pts',(-81.2797370189181,-47.139365595286,173.576925069079));
#46531=CARTESIAN_POINT('Ctrl Pts',(-83.4579294386781,-51.8125322088705,
177.705885069079));
#46532=CARTESIAN_POINT('Ctrl Pts',(-83.4579294386781,-51.8125322088705,
173.576925069079));
#46533=CARTESIAN_POINT('Ctrl Pts',(-84.8050389597313,-55.0309990672248,
177.705885069079));
#46534=CARTESIAN_POINT('Ctrl Pts',(-84.8050389597313,-55.0309990672248,
173.576925069079));
#46535=CARTESIAN_POINT('Ctrl Pts',(-88.5443259067898,-64.7535560405655,
177.705885069079));
#46536=CARTESIAN_POINT('Ctrl Pts',(-88.5443259067898,-64.7535560405655,
173.576925069079));
#46537=CARTESIAN_POINT('Ctrl Pts',(-90.6342709141923,-71.3245283131479,
177.705885069079));
#46538=CARTESIAN_POINT('Ctrl Pts',(-90.6342709141923,-71.3245283131479,
173.576925069079));
#46539=CARTESIAN_POINT('Ctrl Pts',(-94.0886049589878,-83.3618611533263,
177.705885069079));
#46540=CARTESIAN_POINT('Ctrl Pts',(-94.0886049589878,-83.3618611533263,
173.576925069079));
#46541=CARTESIAN_POINT('Ctrl Pts',(-95.4530208414653,-88.8276309456242,
177.705885069079));
#46542=CARTESIAN_POINT('Ctrl Pts',(-95.4530208414653,-88.8276309456242,
173.576925069079));
#46543=CARTESIAN_POINT('Ctrl Pts',(-97.0209399293013,-95.2453104772289,
177.705885069079));
#46544=CARTESIAN_POINT('Ctrl Pts',(-97.0209399293013,-95.2453104772289,
173.576925069079));
#46545=CARTESIAN_POINT('Ctrl Pts',(-97.4636939970592,-97.0873928564593,
177.705885069079));
#46546=CARTESIAN_POINT('Ctrl Pts',(-97.4636939970592,-97.0873928564593,
173.576925069079));
#46547=CARTESIAN_POINT('Ctrl Pts',(-98.0183678164048,-99.2934349167345,
177.705885069079));
#46548=CARTESIAN_POINT('Ctrl Pts',(-98.0183678164048,-99.2934349167345,
173.576925069079));
#46549=CARTESIAN_POINT('Ctrl Pts',(-98.1849688704148,-99.9358635919993,
177.705885069079));
#46550=CARTESIAN_POINT('Ctrl Pts',(-98.1849688704148,-99.9358635919993,
173.576925069079));
#46551=CARTESIAN_POINT('Ctrl Pts',(-98.485392535511,-101.02211760146,177.705885069079));
#46552=CARTESIAN_POINT('Ctrl Pts',(-98.485392535511,-101.02211760146,173.576925069079));
#46553=CARTESIAN_POINT('Ctrl Pts',(-98.6178709133345,-101.46363133471,177.705885069079));
#46554=CARTESIAN_POINT('Ctrl Pts',(-98.6178709133345,-101.46363133471,173.576925069079));
#46555=CARTESIAN_POINT('Ctrl Pts',(-98.7431461249941,-101.814198511965,
177.705885069079));
#46556=CARTESIAN_POINT('Ctrl Pts',(-98.7431461249941,-101.814198511965,
173.576925069079));
#46557=CARTESIAN_POINT('',(-85.8357031165434,-57.713668075261,176.685485069079));
#46558=CARTESIAN_POINT('Ctrl Pts',(-77.3304501603129,-39.7397688129298,
176.685485069079));
#46559=CARTESIAN_POINT('Ctrl Pts',(-77.4354809475772,-39.918618205007,176.685485069079));
#46560=CARTESIAN_POINT('Ctrl Pts',(-77.5387174074033,-40.095017410943,176.685485069079));
#46561=CARTESIAN_POINT('Ctrl Pts',(-77.7452188224523,-40.4514138749057,
176.685485069079));
#46562=CARTESIAN_POINT('Ctrl Pts',(-78.0537048438588,-40.988104564515,176.685485069079));
#46563=CARTESIAN_POINT('Ctrl Pts',(-78.7646561081799,-42.2546401779696,
176.685485069079));
#46564=CARTESIAN_POINT('Ctrl Pts',(-79.358919965841,-43.3632613763041,176.685485069079));
#46565=CARTESIAN_POINT('Ctrl Pts',(-80.5274284163852,-45.6074041562991,
176.685485069079));
#46566=CARTESIAN_POINT('Ctrl Pts',(-81.2797370189181,-47.139365595286,176.685485069079));
#46567=CARTESIAN_POINT('Ctrl Pts',(-83.3745257073509,-51.6335950639466,
176.685485069079));
#46568=CARTESIAN_POINT('Ctrl Pts',(-84.6499486695732,-54.6616303374944,
176.685485069079));
#46569=CARTESIAN_POINT('Ctrl Pts',(-85.8357028732072,-57.7136681697975,
176.685485069079));
#46570=CARTESIAN_POINT('',(-86.4935648641623,-59.4333382806591,176.685485069079));
#46571=CARTESIAN_POINT('Ctrl Pts',(-85.8357032382115,-57.7136680279929,
176.685485069079));
#46572=CARTESIAN_POINT('Ctrl Pts',(-85.8575368827931,-57.7698663129345,
176.685485072469));
#46573=CARTESIAN_POINT('Ctrl Pts',(-85.8790685227464,-57.8253736599762,
176.689988619807));
#46574=CARTESIAN_POINT('Ctrl Pts',(-85.9002716509352,-57.8801146319343,
176.698219460949));
#46575=CARTESIAN_POINT('Ctrl Pts',(-85.9074955079205,-57.8987647551209,
176.701023689587));
#46576=CARTESIAN_POINT('Ctrl Pts',(-85.9146812616168,-57.9173259872642,
176.704260100816));
#46577=CARTESIAN_POINT('Ctrl Pts',(-85.9218279524688,-57.9357955500639,
176.707896698839));
#46578=CARTESIAN_POINT('Ctrl Pts',(-85.9473631106758,-58.0017873801117,
176.720890279754));
#46579=CARTESIAN_POINT('Ctrl Pts',(-85.9724206859325,-58.066662896417,176.739132966205));
#46580=CARTESIAN_POINT('Ctrl Pts',(-85.9971566701928,-58.1308157259833,
176.760337228688));
#46581=CARTESIAN_POINT('Ctrl Pts',(-85.9995997074219,-58.1371517484087,
176.762431457166));
#46582=CARTESIAN_POINT('Ctrl Pts',(-86.002039611443,-58.1434807298304,176.764554536289));
#46583=CARTESIAN_POINT('Ctrl Pts',(-86.0044765344927,-58.1498030537245,
176.766704243004));
#46584=CARTESIAN_POINT('Ctrl Pts',(-86.0044947695771,-58.1498503626085,
176.766720328897));
#46585=CARTESIAN_POINT('Ctrl Pts',(-86.004513004512,-58.1498976711649,176.766736416296));
#46586=CARTESIAN_POINT('Ctrl Pts',(-86.0045312392975,-58.1499449793939,
176.7667525052));
#46587=CARTESIAN_POINT('Ctrl Pts',(-86.0316555436731,-58.2203161281954,
176.790684803966));
#46588=CARTESIAN_POINT('Ctrl Pts',(-86.0584159099637,-58.2898750286768,
176.818336470784));
#46589=CARTESIAN_POINT('Ctrl Pts',(-86.0855089993157,-58.3604325361075,
176.841588389785));
#46590=CARTESIAN_POINT('Ctrl Pts',(-86.0855275926271,-58.3604809579648,
176.841604346997));
#46591=CARTESIAN_POINT('Ctrl Pts',(-86.0855461860946,-58.360529380291,176.841620302136));
#46592=CARTESIAN_POINT('Ctrl Pts',(-86.0855647797187,-58.3605778030869,
176.841636255199));
#46593=CARTESIAN_POINT('Ctrl Pts',(-86.0991224819847,-58.3958857048106,
176.853268569574));
#46594=CARTESIAN_POINT('Ctrl Pts',(-86.1128236371906,-58.4316010060895,
176.863656877716));
#46595=CARTESIAN_POINT('Ctrl Pts',(-86.1265739659578,-58.4674794490787,
176.87090073909));
#46596=CARTESIAN_POINT('Ctrl Pts',(-86.1403017396453,-58.5032990395742,
176.878132718138));
#46597=CARTESIAN_POINT('Ctrl Pts',(-86.1540992591418,-58.5393351357888,
176.882147372206));
#46598=CARTESIAN_POINT('Ctrl Pts',(-86.1679922740321,-58.5756563092537,
176.881927610312));
#46599=CARTESIAN_POINT('Ctrl Pts',(-86.1680170995237,-58.575721211724,176.881927217619));
#46600=CARTESIAN_POINT('Ctrl Pts',(-86.1680419253213,-58.5757861151074,
176.881926811406));
#46601=CARTESIAN_POINT('Ctrl Pts',(-86.168066751425,-58.5758510194043,176.881926391667));
#46602=CARTESIAN_POINT('Ctrl Pts',(-86.1819856190064,-58.6122399076145,
176.881691063191));
#46603=CARTESIAN_POINT('Ctrl Pts',(-86.1961417868957,-58.6492857813369,
176.877082885163));
#46604=CARTESIAN_POINT('Ctrl Pts',(-86.209949809353,-58.6854557833995,176.86935105246));
#46605=CARTESIAN_POINT('Ctrl Pts',(-86.2237241681295,-58.721537603725,176.86163806981));
#46606=CARTESIAN_POINT('Ctrl Pts',(-86.2371818936595,-58.7568245986939,
176.851054685034));
#46607=CARTESIAN_POINT('Ctrl Pts',(-86.2505145561711,-58.7918158238361,
176.8393675931));
#46608=CARTESIAN_POINT('Ctrl Pts',(-86.2505443517163,-58.7918940214677,
176.83934147504));
#46609=CARTESIAN_POINT('Ctrl Pts',(-86.2505741466266,-58.7919722175953,
176.839315351477));
#46610=CARTESIAN_POINT('Ctrl Pts',(-86.2506039409043,-58.7920504122243,
176.839289222431));
#46611=CARTESIAN_POINT('Ctrl Pts',(-86.2772947577064,-58.8621000554093,
176.81588185555));
#46612=CARTESIAN_POINT('Ctrl Pts',(-86.3035333311623,-58.9310915384274,
176.788590780995));
#46613=CARTESIAN_POINT('Ctrl Pts',(-86.3301164702189,-59.0011188486079,
176.764983643558));
#46614=CARTESIAN_POINT('Ctrl Pts',(-86.3301422175475,-59.0011866741631,
176.764960778662));
#46615=CARTESIAN_POINT('Ctrl Pts',(-86.3301679651756,-59.0012545006274,
176.76493791724));
#46616=CARTESIAN_POINT('Ctrl Pts',(-86.3301937131039,-59.0013223280029,
176.7649150593));
#46617=CARTESIAN_POINT('Ctrl Pts',(-86.3548279743324,-59.0662159871751,
176.743045786526));
#46618=CARTESIAN_POINT('Ctrl Pts',(-86.3796895393454,-59.1318204739591,
176.72409006409));
#46619=CARTESIAN_POINT('Ctrl Pts',(-86.4048426318501,-59.1983128551758,
176.710356737887));
#46620=CARTESIAN_POINT('Ctrl Pts',(-86.406872472465,-59.2036787534625,176.709248466079));
#46621=CARTESIAN_POINT('Ctrl Pts',(-86.4089042134845,-59.209050439792,176.708174234396));
#46622=CARTESIAN_POINT('Ctrl Pts',(-86.4109378896597,-59.2144280102915,
176.707135274671));
#46623=CARTESIAN_POINT('Ctrl Pts',(-86.432177732687,-59.27059169784,176.696284313379));
#46624=CARTESIAN_POINT('Ctrl Pts',(-86.4537315983723,-59.3276705378626,
176.689177561902));
#46625=CARTESIAN_POINT('Ctrl Pts',(-86.4753675306458,-59.3850540800865,
176.686583816668));
#46626=CARTESIAN_POINT('Ctrl Pts',(-86.4814286020451,-59.4011294560936,
176.685857207116));
#46627=CARTESIAN_POINT('Ctrl Pts',(-86.4874960982682,-59.4172287082636,
176.685485070601));
#46628=CARTESIAN_POINT('Ctrl Pts',(-86.4935648641623,-59.4333382806591,
176.685485069079));
#46629=CARTESIAN_POINT('',(-98.743146025648,-101.814198524563,176.685485069079));
#46630=CARTESIAN_POINT('Ctrl Pts',(-86.4935648641623,-59.433338280659,176.685485069079));
#46631=CARTESIAN_POINT('Ctrl Pts',(-87.7856096728309,-62.8630783211318,
176.685485069079));
#46632=CARTESIAN_POINT('Ctrl Pts',(-88.9767665307843,-66.3330832476407,
176.685485069079));
#46633=CARTESIAN_POINT('Ctrl Pts',(-91.2072333103094,-73.3336959729049,
176.685485069079));
#46634=CARTESIAN_POINT('Ctrl Pts',(-92.2465762119515,-76.8666920983617,
176.68548506908));
#46635=CARTESIAN_POINT('Ctrl Pts',(-94.2061160331528,-83.9673845124857,
176.685485069079));
#46636=CARTESIAN_POINT('Ctrl Pts',(-95.1241782504859,-87.5338958106165,
176.68548506908));
#46637=CARTESIAN_POINT('Ctrl Pts',(-96.449702093816,-92.8970651812464,176.68548506908));
#46638=CARTESIAN_POINT('Ctrl Pts',(-96.8822526521753,-94.687157625756,176.685485069079));
#46639=CARTESIAN_POINT('Ctrl Pts',(-97.5376559351784,-97.3706189117761,
176.685485069079));
#46640=CARTESIAN_POINT('Ctrl Pts',(-97.7569410503841,-98.264897565372,176.685485069079));
#46641=CARTESIAN_POINT('Ctrl Pts',(-98.099506581766,-99.6028376178243,176.685485069079));
#46642=CARTESIAN_POINT('Ctrl Pts',(-98.2159080866078,-100.048253277279,
176.685485069079));
#46643=CARTESIAN_POINT('Ctrl Pts',(-98.4002244375469,-100.713899477402,
176.685485069079));
#46644=CARTESIAN_POINT('Ctrl Pts',(-98.4633004780488,-100.935364010716,
176.685485069079));
#46645=CARTESIAN_POINT('Ctrl Pts',(-98.5960691137325,-101.376605722965,
176.685485069079));
#46646=CARTESIAN_POINT('Ctrl Pts',(-98.6653474496106,-101.596488546345,
176.685485069079));
#46647=CARTESIAN_POINT('Ctrl Pts',(-98.7431461177365,-101.814198491655,
176.685485069079));
#46648=CARTESIAN_POINT('',(-98.743146025648,-101.814198524563,175.285485069079));
#46649=CARTESIAN_POINT('',(-98.7431461249941,-101.814198511965,177.685485069079));
#46650=CARTESIAN_POINT('',(-86.4935648641564,-59.4333382806435,175.285485069079));
#46651=CARTESIAN_POINT('Ctrl Pts',(-98.7431461177365,-101.814198491655,
175.285485069079));
#46652=CARTESIAN_POINT('Ctrl Pts',(-98.6654638987115,-101.596814414744,
175.285485069079));
#46653=CARTESIAN_POINT('Ctrl Pts',(-98.5962640059336,-101.377220104144,
175.285485069079));
#46654=CARTESIAN_POINT('Ctrl Pts',(-98.4636402639926,-100.936526438504,
175.285485069079));
#46655=CARTESIAN_POINT('Ctrl Pts',(-98.4006272590078,-100.715320031166,
175.285485069079));
#46656=CARTESIAN_POINT('Ctrl Pts',(-98.2164901868202,-100.050423526257,
175.285485069079));
#46657=CARTESIAN_POINT('Ctrl Pts',(-98.100194770959,-99.6054752430948,175.285485069079));
#46658=CARTESIAN_POINT('Ctrl Pts',(-97.7579408317027,-98.2689022351253,
175.285485069079));
#46659=CARTESIAN_POINT('Ctrl Pts',(-97.5388526271146,-97.3754873342376,
175.285485069079));
#46660=CARTESIAN_POINT('Ctrl Pts',(-96.8840551083993,-94.6945997888377,
175.285485069079));
#46661=CARTESIAN_POINT('Ctrl Pts',(-96.451924672254,-92.9061946080142,175.285485069079));
#46662=CARTESIAN_POINT('Ctrl Pts',(-95.1277832686895,-87.5482098153712,
175.285485069079));
#46663=CARTESIAN_POINT('Ctrl Pts',(-94.2107624601005,-83.9851469345354,
175.285485069079));
#46664=CARTESIAN_POINT('Ctrl Pts',(-92.2535686906978,-76.8911105188406,
175.285485069079));
#46665=CARTESIAN_POINT('Ctrl Pts',(-91.2147869939348,-73.3584403924464,
175.285485069079));
#46666=CARTESIAN_POINT('Ctrl Pts',(-88.9819313083959,-66.3482632730971,
175.285485069079));
#46667=CARTESIAN_POINT('Ctrl Pts',(-87.7888733385873,-62.8717417398051,
175.285485069079));
#46668=CARTESIAN_POINT('Ctrl Pts',(-86.4935648641568,-59.4333382806445,
175.285485069079));
#46669=CARTESIAN_POINT('',(-85.8357031165468,-57.7136680752698,175.285485069079));
#46670=CARTESIAN_POINT('Ctrl Pts',(-86.4935648641564,-59.4333382806436,
175.285485069079));
#46671=CARTESIAN_POINT('Ctrl Pts',(-86.4719023592219,-59.3758350423251,
175.285485063649));
#46672=CARTESIAN_POINT('Ctrl Pts',(-86.4502563673306,-59.3184641207399,
175.280747741342));
#46673=CARTESIAN_POINT('Ctrl Pts',(-86.4288596853718,-59.261837956496,175.272056283427));
#46674=CARTESIAN_POINT('Ctrl Pts',(-86.4228645085134,-59.2459717642467,
175.269621007366));
#46675=CARTESIAN_POINT('Ctrl Pts',(-86.4168888826336,-59.2301639886453,
175.266874982765));
#46676=CARTESIAN_POINT('Ctrl Pts',(-86.4109378971216,-59.2144280300232,
175.263834747309));
#46677=CARTESIAN_POINT('Ctrl Pts',(-86.3857421845665,-59.1478039911273,
175.250962778712));
#46678=CARTESIAN_POINT('Ctrl Pts',(-86.3608432187804,-59.0820822507344,
175.232681904101));
#46679=CARTESIAN_POINT('Ctrl Pts',(-86.3361765285873,-59.0170849735409,
175.211303790484));
#46680=CARTESIAN_POINT('Ctrl Pts',(-86.3341807485036,-59.0118260486385,
175.209574088889));
#46681=CARTESIAN_POINT('Ctrl Pts',(-86.3321864908343,-59.0065718720304,
175.207824086198));
#46682=CARTESIAN_POINT('Ctrl Pts',(-86.3301937223889,-59.0013223524624,
175.206054996239));
#46683=CARTESIAN_POINT('Ctrl Pts',(-86.3301651272193,-59.0012470246425,
175.206029610737));
#46684=CARTESIAN_POINT('Ctrl Pts',(-86.33013653242,-59.0011716979463,175.206004220941));
#46685=CARTESIAN_POINT('Ctrl Pts',(-86.3301079379899,-59.0010963723711,
175.20597882686));
#46686=CARTESIAN_POINT('Ctrl Pts',(-86.3035277119236,-58.9310767632205,
175.182373515954));
#46687=CARTESIAN_POINT('Ctrl Pts',(-86.2772919052129,-58.8620925690934,
175.155085719146));
#46688=CARTESIAN_POINT('Ctrl Pts',(-86.2506039439847,-58.7920504203087,
175.131680888139));
#46689=CARTESIAN_POINT('Ctrl Pts',(-86.2505698616544,-58.7919609717507,
175.131650998588));
#46690=CARTESIAN_POINT('Ctrl Pts',(-86.2505357784962,-58.7918715212319,
175.131621116213));
#46691=CARTESIAN_POINT('Ctrl Pts',(-86.2505016945069,-58.7917820687439,
175.131591241042));
#46692=CARTESIAN_POINT('Ctrl Pts',(-86.2371732362759,-58.7568018984936,
175.119908630803));
#46693=CARTESIAN_POINT('Ctrl Pts',(-86.2237197381054,-58.7215259993151,
175.109329580509));
#46694=CARTESIAN_POINT('Ctrl Pts',(-86.2099498106586,-58.6854557868193,
175.101619067419));
#46695=CARTESIAN_POINT('Ctrl Pts',(-86.1961417905151,-58.6492857908156,
175.093887224206));
#46696=CARTESIAN_POINT('Ctrl Pts',(-86.1819856251605,-58.6122399237039,
175.089279016292));
#46697=CARTESIAN_POINT('Ctrl Pts',(-86.1680667516765,-58.5758510200618,
175.089043628923));
#46698=CARTESIAN_POINT('Ctrl Pts',(-86.1680359710866,-58.5757705486126,
175.089043108381));
#46699=CARTESIAN_POINT('Ctrl Pts',(-86.1680051909672,-58.5756900785675,
175.08904260863));
#46700=CARTESIAN_POINT('Ctrl Pts',(-86.1679744113182,-58.5756096099258,
175.08904212966));
#46701=CARTESIAN_POINT('Ctrl Pts',(-86.1540868127237,-58.5393026268904,
175.088826021142));
#46702=CARTESIAN_POINT('Ctrl Pts',(-86.1402962101565,-58.5032846115629,
175.092840073551));
#46703=CARTESIAN_POINT('Ctrl Pts',(-86.1265739460565,-58.4674793971515,
175.100069105802));
#46704=CARTESIAN_POINT('Ctrl Pts',(-86.1128259344222,-58.4316070002417,
175.107311702123));
#46705=CARTESIAN_POINT('Ctrl Pts',(-86.0991257058918,-58.3958941006902,
175.117698434768));
#46706=CARTESIAN_POINT('Ctrl Pts',(-86.0855647542472,-58.3605777367531,
175.129333653249));
#46707=CARTESIAN_POINT('Ctrl Pts',(-86.0855374412273,-58.3605066063059,
175.129357087663));
#46708=CARTESIAN_POINT('Ctrl Pts',(-86.0855101285278,-58.3604354768277,
175.129380526571));
#46709=CARTESIAN_POINT('Ctrl Pts',(-86.0854828161481,-58.3603643483165,
175.129403969966));
#46710=CARTESIAN_POINT('Ctrl Pts',(-86.0584038496732,-58.2898437056168,
175.152647015424));
#46711=CARTESIAN_POINT('Ctrl Pts',(-86.0316436675509,-58.2202853167348,
175.180295334629));
#46712=CARTESIAN_POINT('Ctrl Pts',(-86.004531204833,-58.1499448899798,175.204217332711));
#46713=CARTESIAN_POINT('Ctrl Pts',(-86.0044869333326,-58.1498300322382,
175.204256394554));
#46714=CARTESIAN_POINT('Ctrl Pts',(-86.0044426609819,-58.149715172646,175.204295447499));
#46715=CARTESIAN_POINT('Ctrl Pts',(-86.0043983877799,-58.1496003112007,
175.204334491534));
#46716=CARTESIAN_POINT('Ctrl Pts',(-85.9772659820254,-58.0792085797364,
175.228262252673));
#46717=CARTESIAN_POINT('Ctrl Pts',(-85.9498440260562,-58.0081989380341,
175.248817356079));
#46718=CARTESIAN_POINT('Ctrl Pts',(-85.9218279496276,-57.9357955427215,
175.263073396718));
#46719=CARTESIAN_POINT('Ctrl Pts',(-85.8983583315347,-57.8751417948294,
175.275015962271));
#46720=CARTESIAN_POINT('Ctrl Pts',(-85.8744536632948,-57.8134637449331,
175.282654209087));
#46721=CARTESIAN_POINT('Ctrl Pts',(-85.8500832601142,-57.7506936916401,
175.284838580227));
#46722=CARTESIAN_POINT('Ctrl Pts',(-85.8453078965934,-57.7383939434387,
175.28526660623));
#46723=CARTESIAN_POINT('Ctrl Pts',(-85.8405146387439,-57.7260522388413,
175.285485068332));
#46724=CARTESIAN_POINT('Ctrl Pts',(-85.8357032382103,-57.7136680279897,
175.285485069079));
#46725=CARTESIAN_POINT('Origin',(71.2336965524492,-1004.00503493024,175.285485069079));
#46726=CARTESIAN_POINT('Ctrl Pts',(-99.7596659041602,-101.966952700553,
174.385485069079));
#46727=CARTESIAN_POINT('Ctrl Pts',(-99.7596659041602,-101.966952700553,
173.385485069079));
#46728=CARTESIAN_POINT('Ctrl Pts',(-98.8225296350236,-102.315916327695,
173.385485069079));
#46729=CARTESIAN_POINT('Ctrl Pts',(-99.7292244094599,-101.885202550819,
174.385485069079));
#46730=CARTESIAN_POINT('Ctrl Pts',(-99.7292244094596,-101.88520255082,173.385485069079));
#46731=CARTESIAN_POINT('Ctrl Pts',(-98.792088140323,-102.234166177962,173.385485069079));
#46732=CARTESIAN_POINT('Ctrl Pts',(-99.6987829147594,-101.803452401085,
174.385485069079));
#46733=CARTESIAN_POINT('Ctrl Pts',(-99.6987829147593,-101.803452401085,
173.385485069079));
#46734=CARTESIAN_POINT('Ctrl Pts',(-98.7616466456226,-102.152416028228,
173.385485069079));
#46735=CARTESIAN_POINT('Ctrl Pts',(-99.6531206727089,-101.680827176485,
174.385485069079));
#46736=CARTESIAN_POINT('Ctrl Pts',(-99.6531206727089,-101.680827176486,
173.385485069079));
#46737=CARTESIAN_POINT('Ctrl Pts',(-98.7159844035723,-102.029790803628,
173.385485069079));
#46738=CARTESIAN_POINT('Ctrl Pts',(-99.6378999253588,-101.639952101619,
174.385485069079));
#46739=CARTESIAN_POINT('Ctrl Pts',(-99.6378999253586,-101.639952101619,
173.385485069079));
#46740=CARTESIAN_POINT('Ctrl Pts',(-98.700763656222,-101.988915728762,173.385485069079));
#46741=CARTESIAN_POINT('Ctrl Pts',(-99.6150688043334,-101.578639489318,
174.385485069079));
#46742=CARTESIAN_POINT('Ctrl Pts',(-99.6150688043334,-101.578639489318,
173.385485069079));
#46743=CARTESIAN_POINT('Ctrl Pts',(-98.6779325351968,-101.927603116461,
173.385485069079));
#46744=CARTESIAN_POINT('Ctrl Pts',(-99.609407429959,-101.563252285373,174.385485069079));
#46745=CARTESIAN_POINT('Ctrl Pts',(-99.6094074304456,-101.563252285196,
173.385485069079));
#46746=CARTESIAN_POINT('Ctrl Pts',(-98.6703932517879,-101.907141939063,
173.385485069079));
#46747=CARTESIAN_POINT('Ctrl Pts',(-99.5964225120462,-101.527488620696,
174.385485069079));
#46748=CARTESIAN_POINT('Ctrl Pts',(-99.5964225115595,-101.527488620872,
173.385485069079));
#46749=CARTESIAN_POINT('Ctrl Pts',(-98.6555115664908,-101.866154114362,
173.385485069079));
#46750=CARTESIAN_POINT('Ctrl Pts',(-99.5899497481367,-101.509428783166,
174.385485069079));
#46751=CARTESIAN_POINT('Ctrl Pts',(-99.5899497485787,-101.509428783009,
173.385485069079));
#46752=CARTESIAN_POINT('Ctrl Pts',(-98.648156867377,-101.845631556315,173.385485069079));
#46753=CARTESIAN_POINT('Ctrl Pts',(-99.5318916024491,-101.345511288159,
174.385485069079));
#46754=CARTESIAN_POINT('Ctrl Pts',(-99.531891598913,-101.345511289411,173.385485069079));
#46755=CARTESIAN_POINT('Ctrl Pts',(-98.5826553075554,-101.660698841608,
173.385485069079));
#46756=CARTESIAN_POINT('Ctrl Pts',(-99.4817965056164,-101.190760589972,
174.385485069079));
#46757=CARTESIAN_POINT('Ctrl Pts',(-99.4817965071391,-101.190760589501,
173.385485069079));
#46758=CARTESIAN_POINT('Ctrl Pts',(-98.5290815182737,-101.494767980892,
173.385485069079));
#46759=CARTESIAN_POINT('Ctrl Pts',(-99.3356133931763,-100.717504207786,
174.385485069079));
#46760=CARTESIAN_POINT('Ctrl Pts',(-99.3356133901308,-100.717504208727,
173.385485069079));
#46761=CARTESIAN_POINT('Ctrl Pts',(-98.3746712206805,-100.994876750151,
173.385485069079));
#46762=CARTESIAN_POINT('Ctrl Pts',(-99.2432304743068,-100.389603655864,
174.385485069079));
#46763=CARTESIAN_POINT('Ctrl Pts',(-99.2432304751161,-100.389603655646,
173.385485069075));
#46764=CARTESIAN_POINT('Ctrl Pts',(-98.2801283097388,-100.658823541833,
173.385485069079));
#46765=CARTESIAN_POINT('Ctrl Pts',(-98.9732428581022,-99.3981138801062,
174.385485069079));
#46766=CARTESIAN_POINT('Ctrl Pts',(-98.9732428564835,-99.3981138805421,
173.385485069089));
#46767=CARTESIAN_POINT('Ctrl Pts',(-98.0048456627939,-99.6478885553121,
173.385485069079));
#46768=CARTESIAN_POINT('Ctrl Pts',(-98.8024390932428,-98.724463698621,174.385485069079));
#46769=CARTESIAN_POINT('Ctrl Pts',(-98.802439093562,-98.7244636985413,173.385485069079));
#46770=CARTESIAN_POINT('Ctrl Pts',(-97.8330538201541,-98.9700312938576,
173.385485069079));
#46771=CARTESIAN_POINT('Ctrl Pts',(-98.2964066418388,-96.6983592678497,
174.385485069079));
#46772=CARTESIAN_POINT('Ctrl Pts',(-98.2964066412002,-96.6983592680092,
173.385485069079));
#46773=CARTESIAN_POINT('Ctrl Pts',(-97.324582902825,-96.9341634882031,173.385485069079));
#46774=CARTESIAN_POINT('Ctrl Pts',(-97.9682125919038,-95.3374251041846,
174.385485069079));
#46775=CARTESIAN_POINT('Ctrl Pts',(-97.9682125920466,-95.3374251041595,
173.385485069079));
#46776=CARTESIAN_POINT('Ctrl Pts',(-96.9964329902176,-95.5733167033208,
173.385485069079));
#46777=CARTESIAN_POINT('Ctrl Pts',(-96.9745721058683,-91.2558483999456,
174.385485069079));
#46778=CARTESIAN_POINT('Ctrl Pts',(-96.9745721055826,-91.2558483999958,
173.385485069079));
#46779=CARTESIAN_POINT('Ctrl Pts',(-96.0032637830826,-91.4936758730623,
173.385485069079));
#46780=CARTESIAN_POINT('Ctrl Pts',(-96.3022773498184,-88.5330308242917,
174.385485069079));
#46781=CARTESIAN_POINT('Ctrl Pts',(-96.3022773498185,-88.5330308242917,
173.385485069079));
#46782=CARTESIAN_POINT('Ctrl Pts',(-95.3324240441395,-88.7768173262609,
173.385485069079));
#46783=CARTESIAN_POINT('Ctrl Pts',(-94.1962497890728,-80.3918582514504,
174.385485069079));
#46784=CARTESIAN_POINT('Ctrl Pts',(-94.1962497890724,-80.3918582514505,
173.385485069079));
#46785=CARTESIAN_POINT('Ctrl Pts',(-93.2315633992081,-80.6556182591984,
173.385485069079));
#46786=CARTESIAN_POINT('Ctrl Pts',(-92.6770445486041,-74.9910315479212,
174.385485069079));
#46787=CARTESIAN_POINT('Ctrl Pts',(-92.6770445486971,-74.9910315478917,
173.385485069079));
#46788=CARTESIAN_POINT('Ctrl Pts',(-91.7172498887648,-75.2726409100276,
173.385485069079));
#46789=CARTESIAN_POINT('Ctrl Pts',(-90.1390857940941,-67.0122253917376,
174.385485069079));
#46790=CARTESIAN_POINT('Ctrl Pts',(-90.1390857940475,-67.0122253917524,
173.385485069079));
#46791=CARTESIAN_POINT('Ctrl Pts',(-89.1895555183278,-67.32610380923,173.385485069079));
#46792=CARTESIAN_POINT('Ctrl Pts',(-89.2499340323246,-64.3720031405279,
174.385485069118));
#46793=CARTESIAN_POINT('Ctrl Pts',(-89.2499340324016,-64.3720031404906,
173.385485069156));
#46794=CARTESIAN_POINT('Ctrl Pts',(-88.3043449817598,-64.6976651653227,
173.385485069079));
#46795=CARTESIAN_POINT('Ctrl Pts',(-87.3656218452655,-59.1388679004802,
174.385485069041));
#46796=CARTESIAN_POINT('Ctrl Pts',(-87.3656218451886,-59.1388679005176,
173.385485069003));
#46797=CARTESIAN_POINT('Ctrl Pts',(-86.4294800240879,-59.490766888681,173.385485069079));
#46798=CARTESIAN_POINT('Ctrl Pts',(-86.3706260282542,-56.5458859385069,
174.385485069079));
#46799=CARTESIAN_POINT('Ctrl Pts',(-86.37062602833,-56.5458859384659,173.385485069079));
#46800=CARTESIAN_POINT('Ctrl Pts',(-85.4399803831464,-56.912233189929,173.385485069079));
#46801=CARTESIAN_POINT('Ctrl Pts',(-84.2471258837627,-51.4188822072724,
174.385485069079));
#46802=CARTESIAN_POINT('Ctrl Pts',(-84.2471258836868,-51.4188822073134,
173.385485069079));
#46803=CARTESIAN_POINT('Ctrl Pts',(-83.3299902505975,-51.8178481908489,
173.385485069079));
#46804=CARTESIAN_POINT('Ctrl Pts',(-83.1189413138823,-48.8847318393425,
174.385485069041));
#46805=CARTESIAN_POINT('Ctrl Pts',(-83.1189413140826,-48.8847318392535,
173.385485069003));
#46806=CARTESIAN_POINT('Ctrl Pts',(-82.209794638272,-49.3018557835574,173.385485069079));
#46807=CARTESIAN_POINT('Ctrl Pts',(-81.2948030758993,-45.1409331067813,
174.385485069099));
#46808=CARTESIAN_POINT('Ctrl Pts',(-81.2948030757991,-45.1409331068258,
173.385485069118));
#46809=CARTESIAN_POINT('Ctrl Pts',(-80.4009251217981,-45.5893940515925,
173.385485069079));
#46810=CARTESIAN_POINT('Ctrl Pts',(-80.6646391351484,-43.9026279540674,
174.385485069099));
#46811=CARTESIAN_POINT('Ctrl Pts',(-80.6646391352473,-43.9026279540145,
173.385485069118));
#46812=CARTESIAN_POINT('Ctrl Pts',(-79.7764072455219,-44.3622244628955,
173.385485069079));
#46813=CARTESIAN_POINT('Ctrl Pts',(-79.6803177277805,-42.0620394131515,
174.38548506907));
#46814=CARTESIAN_POINT('Ctrl Pts',(-79.680317727731,-42.062039413178,173.38548506906));
#46815=CARTESIAN_POINT('Ctrl Pts',(-78.8017030821551,-42.539619264928,173.385485069079));
#46816=CARTESIAN_POINT('Ctrl Pts',(-79.345681744444,-41.4513279672577,174.385485069079));
#46817=CARTESIAN_POINT('Ctrl Pts',(-79.3456817444886,-41.4513279672327,
173.385485069079));
#46818=CARTESIAN_POINT('Ctrl Pts',(-78.4704654251786,-41.9351162622582,
173.385485069079));
#46819=CARTESIAN_POINT('Ctrl Pts',(-78.6621302404233,-40.2360419657214,
174.385485069079));
#46820=CARTESIAN_POINT('Ctrl Pts',(-78.6621302403787,-40.2360419657465,
173.385485069079));
#46821=CARTESIAN_POINT('Ctrl Pts',(-77.7941667579945,-40.7327250772214,
173.385485069079));
#46822=CARTESIAN_POINT('Ctrl Pts',(-78.3097223640001,-39.6300292660079,
174.385485068993));
#46823=CARTESIAN_POINT('Ctrl Pts',(-78.3097223639766,-39.6300292660224,
173.385485068964));
#46824=CARTESIAN_POINT('Ctrl Pts',(-77.4471311115058,-40.1359310914719,
173.38548506908));
#46825=CARTESIAN_POINT('Ctrl Pts',(-77.959578073788,-39.0337936757116,174.385485069079));
#46826=CARTESIAN_POINT('Ctrl Pts',(-77.959578073788,-39.0337936757116,173.38548506908));
#46827=CARTESIAN_POINT('Ctrl Pts',(-77.0972759082386,-39.5401877666021,
173.38548506908));
#46828=CARTESIAN_POINT('Ctrl Pts',(-99.6210548294771,-101.594714864612,
174.385485069079));
#46829=CARTESIAN_POINT('Ctrl Pts',(-99.6210548294771,-101.594714864612,
174.34834857337));
#46830=CARTESIAN_POINT('Ctrl Pts',(-99.618332160695,-101.59351716655,174.311500923249));
#46831=CARTESIAN_POINT('Ctrl Pts',(-99.6131135575374,-101.591164496407,
174.275214504829));
#46832=CARTESIAN_POINT('Ctrl Pts',(-99.6078545210065,-101.58879359794,174.238646941769));
#46833=CARTESIAN_POINT('Ctrl Pts',(-99.6000608571668,-101.585250119418,
174.202649876939));
#46834=CARTESIAN_POINT('Ctrl Pts',(-99.5899798151376,-101.580618616698,
174.167471979048));
#46835=CARTESIAN_POINT('Ctrl Pts',(-99.5798490586212,-101.575964273801,
174.132120601952));
#46836=CARTESIAN_POINT('Ctrl Pts',(-99.5674084825397,-101.570211617946,
174.09759691258));
#46837=CARTESIAN_POINT('Ctrl Pts',(-99.5529219608852,-101.563481236162,
174.06411575878));
#46838=CARTESIAN_POINT('Ctrl Pts',(-99.5383060730445,-101.556690751351,
174.030335614699));
#46839=CARTESIAN_POINT('Ctrl Pts',(-99.5216077299695,-101.54890552263,173.997617041083));
#46840=CARTESIAN_POINT('Ctrl Pts',(-99.5031082972169,-101.540277215404,
173.966136832419));
#46841=CARTESIAN_POINT('Ctrl Pts',(-99.4988154010547,-101.538274968769,
173.958831675078));
#46842=CARTESIAN_POINT('Ctrl Pts',(-99.4944255530036,-101.536227420283,
173.951593007567));
#46843=CARTESIAN_POINT('Ctrl Pts',(-99.4899423300563,-101.534136629017,
173.944422680324));
#46844=CARTESIAN_POINT('Ctrl Pts',(-99.4689599025389,-101.524351285588,
173.910864038825));
#46845=CARTESIAN_POINT('Ctrl Pts',(-99.4461069453536,-101.513608878056,
173.8789021653));
#46846=CARTESIAN_POINT('Ctrl Pts',(-99.4216728421184,-101.502084985449,
173.848538290026));
#46847=CARTESIAN_POINT('Ctrl Pts',(-99.3964631122686,-101.490195282903,
173.817210555774));
#46848=CARTESIAN_POINT('Ctrl Pts',(-99.3695702812386,-101.47747374905,173.787583070185));
#46849=CARTESIAN_POINT('Ctrl Pts',(-99.3412946667283,-101.464066201814,
173.759628630428));
#46850=CARTESIAN_POINT('Ctrl Pts',(-99.3115503206794,-101.449962220996,
173.730222142041));
#46851=CARTESIAN_POINT('Ctrl Pts',(-99.2802758323409,-101.43509917539,173.702666199029));
#46852=CARTESIAN_POINT('Ctrl Pts',(-99.2478012559472,-101.419594345565,
173.676910847654));
#46853=CARTESIAN_POINT('Ctrl Pts',(-99.2256833056099,-101.409034236884,
173.659369261408));
#46854=CARTESIAN_POINT('Ctrl Pts',(-99.2030082431429,-101.398175294163,
173.642662567942));
#46855=CARTESIAN_POINT('Ctrl Pts',(-99.1798756003963,-101.387041827359,
173.626773374128));
#46856=CARTESIAN_POINT('Ctrl Pts',(-99.1494216646984,-101.372384709024,
173.605855379933));
#46857=CARTESIAN_POINT('Ctrl Pts',(-99.1183874733352,-101.357358017017,
173.586499314387));
#46858=CARTESIAN_POINT('Ctrl Pts',(-99.0868248128164,-101.342034097248,
173.568583317232));
#46859=CARTESIAN_POINT('Ctrl Pts',(-99.0545962472609,-101.326386875349,
173.550289330626));
#46860=CARTESIAN_POINT('Ctrl Pts',(-99.0218164572501,-101.310429158371,
173.533496191528));
#46861=CARTESIAN_POINT('Ctrl Pts',(-98.9885233176074,-101.294191619556,
173.518100410703));
#46862=CARTESIAN_POINT('Ctrl Pts',(-98.9544252291626,-101.277561495735,
173.502332396574));
#46863=CARTESIAN_POINT('Ctrl Pts',(-98.9197884262851,-101.260637206904,
173.48802953069));
#46864=CARTESIAN_POINT('Ctrl Pts',(-98.8846392312882,-101.243413123976,
173.475117316581));
#46865=CARTESIAN_POINT('Ctrl Pts',(-98.854532300697,-101.228659890816,173.464057400871));
#46866=CARTESIAN_POINT('Ctrl Pts',(-98.8240491005275,-101.213685789607,
173.454018251898));
#46867=CARTESIAN_POINT('Ctrl Pts',(-98.7932002122912,-101.198471277188,
173.444978177844));
#46868=CARTESIAN_POINT('Ctrl Pts',(-98.7399202961621,-101.172193897612,
173.429364831143));
#46869=CARTESIAN_POINT('Ctrl Pts',(-98.6859976032515,-101.145478653186,
173.4168867974));
#46870=CARTESIAN_POINT('Ctrl Pts',(-98.6317552693108,-101.118520958096,
173.407465229906));
#46871=CARTESIAN_POINT('Ctrl Pts',(-98.5731330334416,-101.089386511894,
173.397282899762));
#46872=CARTESIAN_POINT('Ctrl Pts',(-98.5141370068313,-101.059967683379,
173.390669338173));
#46873=CARTESIAN_POINT('Ctrl Pts',(-98.4551572085075,-101.030463121763,
173.387558540043));
#46874=CARTESIAN_POINT('Ctrl Pts',(-98.4289295637809,-101.017342779173,
173.386175203537));
#46875=CARTESIAN_POINT('Ctrl Pts',(-98.4027049473097,-101.004204997354,
173.385485069079));
#46876=CARTESIAN_POINT('Ctrl Pts',(-98.3765170572744,-100.991065637145,
173.385485069079));
#46877=CARTESIAN_POINT('Ctrl Pts',(-77.959578073788,-39.0337936757116,177.585485069079));
#46878=CARTESIAN_POINT('Ctrl Pts',(-77.959578073788,-39.0337936757116,178.585485069079));
#46879=CARTESIAN_POINT('Ctrl Pts',(-77.0972759082386,-39.5401877666022,
178.585485069079));
#46880=CARTESIAN_POINT('Ctrl Pts',(-78.3097223640055,-39.6300292660171,
177.585485069079));
#46881=CARTESIAN_POINT('Ctrl Pts',(-78.3097223640027,-39.6300292660199,
178.585485069079));
#46882=CARTESIAN_POINT('Ctrl Pts',(-77.4471311115041,-40.1359310914853,
178.585485069079));
#46883=CARTESIAN_POINT('Ctrl Pts',(-78.6621302404163,-40.2360419657091,
177.585485069108));
#46884=CARTESIAN_POINT('Ctrl Pts',(-78.6621302403905,-40.2360419657227,
178.585485069118));
#46885=CARTESIAN_POINT('Ctrl Pts',(-77.7941667579824,-40.7327250772121,
178.585485069079));
#46886=CARTESIAN_POINT('Ctrl Pts',(-79.345681744451,-41.4513279672701,177.585485069051));
#46887=CARTESIAN_POINT('Ctrl Pts',(-79.3456817444768,-41.4513279672565,
178.585485069041));
#46888=CARTESIAN_POINT('Ctrl Pts',(-78.4704654251907,-41.9351162622676,
178.585485069079));
#46889=CARTESIAN_POINT('Ctrl Pts',(-79.6803177277905,-42.0620394131701,
177.58548506907));
#46890=CARTESIAN_POINT('Ctrl Pts',(-79.6803177277355,-42.0620394131988,
178.58548506906));
#46891=CARTESIAN_POINT('Ctrl Pts',(-78.8017030821739,-42.5396192649393,
178.585485069079));
#46892=CARTESIAN_POINT('Ctrl Pts',(-80.6646391351287,-43.9026279540306,
177.585485069099));
#46893=CARTESIAN_POINT('Ctrl Pts',(-80.6646391352386,-43.9026279539731,
178.585485069118));
#46894=CARTESIAN_POINT('Ctrl Pts',(-79.7764072454845,-44.3622244628733,
178.585485069079));
#46895=CARTESIAN_POINT('Ctrl Pts',(-81.2948030758967,-45.1409331067761,
177.585485069079));
#46896=CARTESIAN_POINT('Ctrl Pts',(-81.2948030758329,-45.1409331068024,
178.585485069079));
#46897=CARTESIAN_POINT('Ctrl Pts',(-80.4009251217938,-45.5893940515883,
178.585485069079));
#46898=CARTESIAN_POINT('Ctrl Pts',(-83.1189413138873,-48.8847318393527,
177.585485069079));
#46899=CARTESIAN_POINT('Ctrl Pts',(-83.1189413140149,-48.8847318393001,
178.585485069079));
#46900=CARTESIAN_POINT('Ctrl Pts',(-82.2097946382807,-49.3018557835656,
178.585485069079));
#46901=CARTESIAN_POINT('Ctrl Pts',(-84.2471258837835,-51.4188822073225,
177.585485069079));
#46902=CARTESIAN_POINT('Ctrl Pts',(-84.2471258836941,-51.41888220735,178.585485069079));
#46903=CARTESIAN_POINT('Ctrl Pts',(-83.3299902506047,-51.8178481909141,
178.585485069079));
#46904=CARTESIAN_POINT('Ctrl Pts',(-86.3706260282335,-56.5458859384568,
177.585485069079));
#46905=CARTESIAN_POINT('Ctrl Pts',(-86.3706260283228,-56.5458859384294,
178.585485069079));
#46906=CARTESIAN_POINT('Ctrl Pts',(-85.4399803831393,-56.9122331898639,
178.585485069079));
#46907=CARTESIAN_POINT('Ctrl Pts',(-87.3656218452865,-59.1388679005385,
177.585485069041));
#46908=CARTESIAN_POINT('Ctrl Pts',(-87.3656218451422,-59.1388679005916,
178.585485069003));
#46909=CARTESIAN_POINT('Ctrl Pts',(-86.4294800241184,-59.490766888736,178.585485069079));
#46910=CARTESIAN_POINT('Ctrl Pts',(-89.2499340323036,-64.3720031404696,
177.585485069118));
#46911=CARTESIAN_POINT('Ctrl Pts',(-89.2499340324479,-64.3720031404165,
178.585485069156));
#46912=CARTESIAN_POINT('Ctrl Pts',(-88.3043449817293,-64.6976651652677,
178.585485069079));
#46913=CARTESIAN_POINT('Ctrl Pts',(-90.1390857941228,-67.0122253918278,
177.585485069079));
#46914=CARTESIAN_POINT('Ctrl Pts',(-90.1390857940778,-67.0122253918421,
178.585485069079));
#46915=CARTESIAN_POINT('Ctrl Pts',(-89.1895555183389,-67.3261038093198,
178.585485069079));
#46916=CARTESIAN_POINT('Ctrl Pts',(-92.6770445485467,-74.9910315477408,
177.585485069079));
#46917=CARTESIAN_POINT('Ctrl Pts',(-92.6770445486365,-74.9910315477122,
178.585485069079));
#46918=CARTESIAN_POINT('Ctrl Pts',(-91.7172498887427,-75.272640909848,178.585485069079));
#46919=CARTESIAN_POINT('Ctrl Pts',(-94.1962497890392,-80.3918582513208,
177.585485069079));
#46920=CARTESIAN_POINT('Ctrl Pts',(-94.1962497890132,-80.3918582513275,
178.585485069002));
#46921=CARTESIAN_POINT('Ctrl Pts',(-93.2315633991488,-80.6556182590752,
178.585485069079));
#46922=CARTESIAN_POINT('Ctrl Pts',(-96.3022773498351,-88.5330308243565,
177.585485069079));
#46923=CARTESIAN_POINT('Ctrl Pts',(-96.3022773498481,-88.5330308243531,
178.585485069118));
#46924=CARTESIAN_POINT('Ctrl Pts',(-95.3324240441691,-88.7768173263224,
178.585485069079));
#46925=CARTESIAN_POINT('Ctrl Pts',(-96.974572105871,-91.2558483999567,177.585485069079));
#46926=CARTESIAN_POINT('Ctrl Pts',(-96.9745721056358,-91.2558483999945,
178.585485069079));
#46927=CARTESIAN_POINT('Ctrl Pts',(-96.0032637831359,-91.4936758730611,
178.585485069079));
#46928=CARTESIAN_POINT('Ctrl Pts',(-97.9682125919025,-95.3374251041791,
177.585485069079));
#46929=CARTESIAN_POINT('Ctrl Pts',(-97.96821259202,-95.3374251041602,178.585485069079));
#46930=CARTESIAN_POINT('Ctrl Pts',(-96.996432990191,-95.5733167033214,178.585485069079));
#46931=CARTESIAN_POINT('Ctrl Pts',(-98.2964066418423,-96.6983592678637,
177.585485069079));
#46932=CARTESIAN_POINT('Ctrl Pts',(-98.2964066411991,-96.6983592680243,
178.585485069079));
#46933=CARTESIAN_POINT('Ctrl Pts',(-97.3245829028239,-96.9341634882086,
178.585485069079));
#46934=CARTESIAN_POINT('Ctrl Pts',(-98.802439093241,-98.724463698614,177.585485069079));
#46935=CARTESIAN_POINT('Ctrl Pts',(-98.8024390935625,-98.7244636985337,
178.585485069079));
#46936=CARTESIAN_POINT('Ctrl Pts',(-97.8330538201546,-98.9700312938548,
178.585485069079));
#46937=CARTESIAN_POINT('Ctrl Pts',(-98.9732428581051,-99.3981138801168,
177.585485069079));
#46938=CARTESIAN_POINT('Ctrl Pts',(-98.9732428564852,-99.3981138805579,
178.585485069079));
#46939=CARTESIAN_POINT('Ctrl Pts',(-98.0048456627956,-99.6478885553231,
178.585485069079));
#46940=CARTESIAN_POINT('Ctrl Pts',(-99.2432304743053,-100.389603655859,
177.585485069079));
#46941=CARTESIAN_POINT('Ctrl Pts',(-99.2432304751152,-100.389603655638,
178.585485069079));
#46942=CARTESIAN_POINT('Ctrl Pts',(-98.2801283097379,-100.658823541827,
178.585485069079));
#46943=CARTESIAN_POINT('Ctrl Pts',(-99.3356133931767,-100.717504207787,
177.585485069079));
#46944=CARTESIAN_POINT('Ctrl Pts',(-99.3356133901333,-100.717504208727,
178.585485069079));
#46945=CARTESIAN_POINT('Ctrl Pts',(-98.3746712206855,-100.994876750151,
178.585485069079));
#46946=CARTESIAN_POINT('Ctrl Pts',(-99.4817965056161,-101.190760589971,
177.585485069079));
#46947=CARTESIAN_POINT('Ctrl Pts',(-99.4817965071378,-101.190760589501,
178.585485069079));
#46948=CARTESIAN_POINT('Ctrl Pts',(-98.5290815182711,-101.494767980891,
178.585485069079));
#46949=CARTESIAN_POINT('Ctrl Pts',(-99.5318916024483,-101.345511288157,
177.585485069079));
#46950=CARTESIAN_POINT('Ctrl Pts',(-99.5318915989119,-101.345511289408,
178.585485069079));
#46951=CARTESIAN_POINT('Ctrl Pts',(-98.5826553075542,-101.660698841605,
178.585485069079));
#46952=CARTESIAN_POINT('Ctrl Pts',(-99.5899497481368,-101.509428783166,
177.585485069079));
#46953=CARTESIAN_POINT('Ctrl Pts',(-99.5899497485788,-101.50942878301,178.585485069079));
#46954=CARTESIAN_POINT('Ctrl Pts',(-98.6481568673771,-101.845631556315,
178.585485069079));
#46955=CARTESIAN_POINT('Ctrl Pts',(-99.5964225120462,-101.527488620696,
177.585485069079));
#46956=CARTESIAN_POINT('Ctrl Pts',(-99.5964225115594,-101.527488620873,
178.585485069079));
#46957=CARTESIAN_POINT('Ctrl Pts',(-98.6555115664906,-101.866154114362,
178.585485069079));
#46958=CARTESIAN_POINT('Ctrl Pts',(-99.6094074299589,-101.563252285373,
177.585485069079));
#46959=CARTESIAN_POINT('Ctrl Pts',(-99.6094074304457,-101.563252285196,
178.585485069079));
#46960=CARTESIAN_POINT('Ctrl Pts',(-98.6703932517879,-101.907141939062,
178.585485069079));
#46961=CARTESIAN_POINT('Ctrl Pts',(-99.6150688043333,-101.578639489318,
177.585485069079));
#46962=CARTESIAN_POINT('Ctrl Pts',(-99.6150688043334,-101.578639489318,
178.585485069079));
#46963=CARTESIAN_POINT('Ctrl Pts',(-98.6779325351968,-101.927603116461,
178.585485069079));
#46964=CARTESIAN_POINT('Ctrl Pts',(-99.6378999253588,-101.639952101619,
177.585485069079));
#46965=CARTESIAN_POINT('Ctrl Pts',(-99.6378999253585,-101.639952101619,
178.585485069079));
#46966=CARTESIAN_POINT('Ctrl Pts',(-98.7007636562219,-101.988915728762,
178.585485069079));
#46967=CARTESIAN_POINT('Ctrl Pts',(-99.6531206727089,-101.680827176486,
177.585485069079));
#46968=CARTESIAN_POINT('Ctrl Pts',(-99.653120672709,-101.680827176486,178.585485069079));
#46969=CARTESIAN_POINT('Ctrl Pts',(-98.7159844035723,-102.029790803628,
178.585485069079));
#46970=CARTESIAN_POINT('Ctrl Pts',(-99.6987829147594,-101.803452401085,
177.585485069079));
#46971=CARTESIAN_POINT('Ctrl Pts',(-99.6987829147592,-101.803452401085,
178.585485069079));
#46972=CARTESIAN_POINT('Ctrl Pts',(-98.7616466456226,-102.152416028228,
178.585485069079));
#46973=CARTESIAN_POINT('Ctrl Pts',(-99.7292244094599,-101.885202550819,
177.585485069079));
#46974=CARTESIAN_POINT('Ctrl Pts',(-99.7292244094612,-101.885202550819,
178.585485069079));
#46975=CARTESIAN_POINT('Ctrl Pts',(-98.7920881403248,-102.234166177961,
178.585485069079));
#46976=CARTESIAN_POINT('Ctrl Pts',(-99.7596659041602,-101.966952700553,
177.585485069079));
#46977=CARTESIAN_POINT('Ctrl Pts',(-99.7596659041602,-101.966952700553,
178.585485069079));
#46978=CARTESIAN_POINT('Ctrl Pts',(-98.8225296350236,-102.315916327695,
178.585485069079));
#46979=CARTESIAN_POINT('Ctrl Pts',(-98.3765170572744,-100.991065637145,
178.585485069079));
#46980=CARTESIAN_POINT('Ctrl Pts',(-98.4305822075695,-101.018191972391,
178.585485069079));
#46981=CARTESIAN_POINT('Ctrl Pts',(-98.4847274747232,-101.045274025794,
178.582547152259));
#46982=CARTESIAN_POINT('Ctrl Pts',(-98.5387005379516,-101.07219166779,178.576651720296));
#46983=CARTESIAN_POINT('Ctrl Pts',(-98.5902438653333,-101.097897543106,
178.571021686322));
#46984=CARTESIAN_POINT('Ctrl Pts',(-98.641630625025,-101.123454767852,178.562693776218));
#46985=CARTESIAN_POINT('Ctrl Pts',(-98.6926335233544,-101.148738472462,
178.551610199999));
#46986=CARTESIAN_POINT('Ctrl Pts',(-98.7263492605821,-101.16545239988,178.544283342985));
#46987=CARTESIAN_POINT('Ctrl Pts',(-98.7598970862398,-101.182046353722,
178.535751434339));
#46988=CARTESIAN_POINT('Ctrl Pts',(-98.7932079208523,-101.19847507901,178.525989701346));
#46989=CARTESIAN_POINT('Ctrl Pts',(-98.8292147103055,-101.216233434791,
178.51543791936));
#46990=CARTESIAN_POINT('Ctrl Pts',(-98.8647234933833,-101.233664780123,
178.503526033788));
#46991=CARTESIAN_POINT('Ctrl Pts',(-98.8997168217397,-101.250798523256,
178.490216331959));
#46992=CARTESIAN_POINT('Ctrl Pts',(-98.934244743073,-101.267704389684,178.477083647549));
#46993=CARTESIAN_POINT('Ctrl Pts',(-98.9682710919285,-101.284321222224,
178.462589629479));
#46994=CARTESIAN_POINT('Ctrl Pts',(-99.0017689542116,-101.300650006337,
178.446657516942));
#46995=CARTESIAN_POINT('Ctrl Pts',(-99.0341907378252,-101.316454247834,
178.431237204421));
#46996=CARTESIAN_POINT('Ctrl Pts',(-99.0661176319256,-101.331989156102,
178.414469133947));
#46997=CARTESIAN_POINT('Ctrl Pts',(-99.0975124519308,-101.347221299307,
178.396253114668));
#46998=CARTESIAN_POINT('Ctrl Pts',(-99.1254005310773,-101.360752041486,
178.380071789617));
#46999=CARTESIAN_POINT('Ctrl Pts',(-99.1528687077778,-101.37404373471,178.362747252573));
#47000=CARTESIAN_POINT('Ctrl Pts',(-99.1798801448296,-101.387044014541,
178.344193642566));
#47001=CARTESIAN_POINT('Ctrl Pts',(-99.2137741126018,-101.403356773642,
178.320912561354));
#47002=CARTESIAN_POINT('Ctrl Pts',(-99.2466864709949,-101.419082201428,
178.295876339252));
#47003=CARTESIAN_POINT('Ctrl Pts',(-99.2783014428484,-101.43413658413,178.26903067634));
#47004=CARTESIAN_POINT('Ctrl Pts',(-99.3088775986878,-101.448696304559,
178.24306711779));
#47005=CARTESIAN_POINT('Ctrl Pts',(-99.338240285646,-101.462628511189,178.215410332517));
#47006=CARTESIAN_POINT('Ctrl Pts',(-99.3660875946641,-101.475813840283,
178.186019035509));
#47007=CARTESIAN_POINT('Ctrl Pts',(-99.3925585906586,-101.488347503532,
178.158080360901));
#47008=CARTESIAN_POINT('Ctrl Pts',(-99.4176602614692,-101.500206193845,
178.12857375169));
#47009=CARTESIAN_POINT('Ctrl Pts',(-99.4411182957459,-101.511247128345,
178.097480701142));
#47010=CARTESIAN_POINT('Ctrl Pts',(-99.4583148829155,-101.519341003149,
178.074687045552));
#47011=CARTESIAN_POINT('Ctrl Pts',(-99.4746278674543,-101.526994593327,
178.051041097961));
#47012=CARTESIAN_POINT('Ctrl Pts',(-99.4899438535657,-101.534137339519,
178.026545021173));
#47013=CARTESIAN_POINT('Ctrl Pts',(-99.5101721875391,-101.543571002779,
177.994192235091));
#47014=CARTESIAN_POINT('Ctrl Pts',(-99.5284988040617,-101.552122304806,
177.960443704363));
#47015=CARTESIAN_POINT('Ctrl Pts',(-99.5445987150435,-101.559611735255,
177.9254913044));
#47016=CARTESIAN_POINT('Ctrl Pts',(-99.5598249635931,-101.566694751405,
177.892435598076));
#47017=CARTESIAN_POINT('Ctrl Pts',(-99.5730594840834,-101.572827664698,
177.858303807702));
#47018=CARTESIAN_POINT('Ctrl Pts',(-99.5840370353095,-101.577884571358,
177.823302561404));
#47019=CARTESIAN_POINT('Ctrl Pts',(-99.5949550980474,-101.582914074116,
177.788490990489));
#47020=CARTESIAN_POINT('Ctrl Pts',(-99.6036404116704,-101.586878730474,
177.752819756212));
#47021=CARTESIAN_POINT('Ctrl Pts',(-99.6098441942121,-101.589687356005,
177.716529959633));
#47022=CARTESIAN_POINT('Ctrl Pts',(-99.6160114909652,-101.592479463401,
177.680453591207));
#47023=CARTESIAN_POINT('Ctrl Pts',(-99.6197262175262,-101.594128716056,
177.643766413933));
#47024=CARTESIAN_POINT('Ctrl Pts',(-99.620758383797,-101.594584275658,177.606736088151));
#47025=CARTESIAN_POINT('Ctrl Pts',(-99.6209555024414,-101.594671276458,
177.599664196899));
#47026=CARTESIAN_POINT('Ctrl Pts',(-99.621054829477,-101.594714864612,177.592579867853));
#47027=CARTESIAN_POINT('Ctrl Pts',(-99.621054829477,-101.594714864612,177.585485069079));
#47028=CARTESIAN_POINT('Origin',(-99.2720912023343,-100.657578595475,174.385485069079));
#47029=CARTESIAN_POINT('Origin',(-98.8390996009298,-100.81881269208,174.385485069078));
#47030=CARTESIAN_POINT('Origin',(-101.649120271255,-99.7724387145074,177.585485069079));
#47031=CARTESIAN_POINT('Origin',(-98.839099600931,-100.818812692077,177.585485069078));
#47032=CARTESIAN_POINT('Origin',(-98.8390996009304,-100.818812692078,173.835485069079));
#47033=CARTESIAN_POINT('Ctrl Pts',(-97.8838106717875,-101.114486603435,
174.36571584829));
#47034=CARTESIAN_POINT('Ctrl Pts',(-97.8849135881754,-101.118050001404,
174.365742603133));
#47035=CARTESIAN_POINT('Ctrl Pts',(-97.8860364212679,-101.121607157985,
174.365777961194));
#47036=CARTESIAN_POINT('Ctrl Pts',(-97.8885814335997,-101.129515393127,
174.365875899567));
#47037=CARTESIAN_POINT('Ctrl Pts',(-97.8900136419527,-101.133863154473,
174.365942839133));
#47038=CARTESIAN_POINT('Ctrl Pts',(-97.895926912204,-101.151407824776,174.366266229089));
#47039=CARTESIAN_POINT('Ctrl Pts',(-97.9006535276767,-101.164519262059,
174.366630166537));
#47040=CARTESIAN_POINT('Ctrl Pts',(-97.9353481098766,-101.254802793895,
174.370007852721));
#47041=CARTESIAN_POINT('Ctrl Pts',(-97.9745478504433,-101.327964563021,
174.377064983029));
#47042=CARTESIAN_POINT('Ctrl Pts',(-98.0731118853643,-101.467848500997,
174.403591185806));
#47043=CARTESIAN_POINT('Ctrl Pts',(-98.1332873077329,-101.532286752824,
174.423968754122));
#47044=CARTESIAN_POINT('Ctrl Pts',(-98.2601167611847,-101.638089049953,
174.48329793291));
#47045=CARTESIAN_POINT('Ctrl Pts',(-98.3243130154484,-101.67900994078,174.520374455133));
#47046=CARTESIAN_POINT('Ctrl Pts',(-98.45418690728,-101.744830959462,174.61988553992));
#47047=CARTESIAN_POINT('Ctrl Pts',(-98.5164960369575,-101.766963654996,
174.681676275863));
#47048=CARTESIAN_POINT('Ctrl Pts',(-98.6272597346526,-101.797936714345,
174.83240435999));
#47049=CARTESIAN_POINT('Ctrl Pts',(-98.6719708237926,-101.805199932678,
174.920075475286));
#47050=CARTESIAN_POINT('Ctrl Pts',(-98.7291347063541,-101.813138240831,
175.101678439926));
#47051=CARTESIAN_POINT('Ctrl Pts',(-98.7431458989486,-101.814198490187,
175.193418679837));
#47052=CARTESIAN_POINT('Ctrl Pts',(-98.7431458989518,-101.814198490187,
175.285485069079));
#47053=CARTESIAN_POINT('Ctrl Pts',(-98.7431458989518,-101.814198490187,
176.685485069079));
#47054=CARTESIAN_POINT('Ctrl Pts',(-98.7431458989486,-101.814198490187,
176.776650914172));
#47055=CARTESIAN_POINT('Ctrl Pts',(-98.7294079789718,-101.813153557324,
176.867502767005));
#47056=CARTESIAN_POINT('Ctrl Pts',(-98.6730268299348,-101.805370421282,
177.048509953544));
#47057=CARTESIAN_POINT('Ctrl Pts',(-98.6285238159208,-101.798198724887,
177.136402953419));
#47058=CARTESIAN_POINT('Ctrl Pts',(-98.5180661808909,-101.767485380609,
177.287557268415));
#47059=CARTESIAN_POINT('Ctrl Pts',(-98.4558597070305,-101.745515778251,
177.349562701941));
#47060=CARTESIAN_POINT('Ctrl Pts',(-98.3258752989752,-101.67995039206,177.449617759738));
#47061=CARTESIAN_POINT('Ctrl Pts',(-98.2614711785115,-101.639064877108,
177.486951211427));
#47062=CARTESIAN_POINT('Ctrl Pts',(-98.1344522768478,-101.533418132759,
177.546546970785));
#47063=CARTESIAN_POINT('Ctrl Pts',(-98.0742734413384,-101.469197196162,
177.567003050164));
#47064=CARTESIAN_POINT('Ctrl Pts',(-97.9752073410398,-101.329171021278,
177.593784778556));
#47065=CARTESIAN_POINT('Ctrl Pts',(-97.9356541020267,-101.255545406551,
177.600926124503));
#47066=CARTESIAN_POINT('Ctrl Pts',(-97.900713297569,-101.164683712518,177.604335211391));
#47067=CARTESIAN_POINT('Ctrl Pts',(-97.8959658633087,-101.151520598178,
177.60470145546));
#47068=CARTESIAN_POINT('Ctrl Pts',(-97.8900295966086,-101.133911400201,
177.605026531602));
#47069=CARTESIAN_POINT('Ctrl Pts',(-97.8885931810068,-101.129551518366,
177.605093742951));
#47070=CARTESIAN_POINT('Ctrl Pts',(-97.8860414703018,-101.121623153065,
177.605192017933));
#47071=CARTESIAN_POINT('Ctrl Pts',(-97.8849160678685,-101.118058013011,
177.605227474873));
#47072=CARTESIAN_POINT('Ctrl Pts',(-97.8838106717876,-101.114486603435,
177.605254289869));
#47073=CARTESIAN_POINT('Ctrl Pts',(-97.8932302579351,-102.399362986829,
177.685485069079));
#47074=CARTESIAN_POINT('Ctrl Pts',(-98.8303665270718,-102.050399359687,
177.685485069079));
#47075=CARTESIAN_POINT('Ctrl Pts',(-98.8303665270718,-102.050399359687,
176.685485069079));
#47076=CARTESIAN_POINT('Ctrl Pts',(-97.8730369312331,-102.34513412923,177.685485069079));
#47077=CARTESIAN_POINT('Ctrl Pts',(-98.8109710951273,-101.998313235765,
177.685485069079));
#47078=CARTESIAN_POINT('Ctrl Pts',(-98.8109710951313,-101.998313235766,
176.685485069079));
#47079=CARTESIAN_POINT('Ctrl Pts',(-97.8527181088294,-102.290940987051,
177.685485069079));
#47080=CARTESIAN_POINT('Ctrl Pts',(-98.7883769389248,-101.937964302332,
177.685485069079));
#47081=CARTESIAN_POINT('Ctrl Pts',(-98.7883769378891,-101.937964302715,
176.685485069079));
#47082=CARTESIAN_POINT('Ctrl Pts',(-97.8126362132817,-102.182375180482,
177.685485069079));
#47083=CARTESIAN_POINT('Ctrl Pts',(-98.7531924801363,-101.842663688618,
177.685485069079));
#47084=CARTESIAN_POINT('Ctrl Pts',(-98.7531924811721,-101.842663688236,
176.685485069079));
#47085=CARTESIAN_POINT('Ctrl Pts',(-97.7931741603528,-102.127898788951,
177.685485069079));
#47086=CARTESIAN_POINT('Ctrl Pts',(-98.7358013339773,-101.794005894027,
177.685485069079));
#47087=CARTESIAN_POINT('Ctrl Pts',(-98.7358013331175,-101.794005894326,
176.685485069079));
#47088=CARTESIAN_POINT('Ctrl Pts',(-97.7361407722699,-101.964017467933,
177.685485069079));
#47089=CARTESIAN_POINT('Ctrl Pts',(-98.6842094799426,-101.645760425827,
177.685485069079));
#47090=CARTESIAN_POINT('Ctrl Pts',(-98.6842094816623,-101.645760425228,
176.685485069079));
#47091=CARTESIAN_POINT('Ctrl Pts',(-97.6999002805471,-101.854167720931,
177.685485069079));
#47092=CARTESIAN_POINT('Ctrl Pts',(-98.6505921303461,-101.54395040367,177.685485069079));
#47093=CARTESIAN_POINT('Ctrl Pts',(-98.6505921292553,-101.543950404017,
176.685485069079));
#47094=CARTESIAN_POINT('Ctrl Pts',(-97.5945716173814,-101.523484475616,
177.685485069079));
#47095=CARTESIAN_POINT('Ctrl Pts',(-98.5516872373819,-101.233434821501,
177.685485069079));
#47096=CARTESIAN_POINT('Ctrl Pts',(-98.5516872395635,-101.233434820807,
176.685485069079));
#47097=CARTESIAN_POINT('Ctrl Pts',(-97.5287765043858,-101.301550314339,
177.685485069079));
#47098=CARTESIAN_POINT('Ctrl Pts',(-98.4883057294024,-101.019857554285,
177.685485069079));
#47099=CARTESIAN_POINT('Ctrl Pts',(-98.4883057284991,-101.019857554543,
176.685485069079));
#47100=CARTESIAN_POINT('Ctrl Pts',(-97.337669387055,-100.633649414688,177.685485069079));
#47101=CARTESIAN_POINT('Ctrl Pts',(-98.3028651239191,-100.371760565047,
177.685485069079));
#47102=CARTESIAN_POINT('Ctrl Pts',(-98.3028651257257,-100.37176056453,176.685485069079));
#47103=CARTESIAN_POINT('Ctrl Pts',(-97.2185417746632,-100.185615621848,
177.685485069079));
#47104=CARTESIAN_POINT('Ctrl Pts',(-98.1852802927309,-99.9298032981305,
177.685485069079));
#47105=CARTESIAN_POINT('Ctrl Pts',(-98.1852802922409,-99.9298032982608,
176.685485069079));
#47106=CARTESIAN_POINT('Ctrl Pts',(-96.8691183172638,-98.8388539217306,
177.685485069079));
#47107=CARTESIAN_POINT('Ctrl Pts',(-97.8394941595671,-98.5970607167195,
177.685485069079));
#47108=CARTESIAN_POINT('Ctrl Pts',(-97.839494160547,-98.5970607164588,176.685485069079));
#47109=CARTESIAN_POINT('Ctrl Pts',(-96.6472483679273,-97.9373097658594,
177.685485069079));
#47110=CARTESIAN_POINT('Ctrl Pts',(-97.6181791273144,-97.6979435767543,
177.685485069079));
#47111=CARTESIAN_POINT('Ctrl Pts',(-97.6181791271038,-97.6979435768059,
176.685485069079));
#47112=CARTESIAN_POINT('Ctrl Pts',(-95.9849221665839,-95.2315797811142,
177.685485069079));
#47113=CARTESIAN_POINT('Ctrl Pts',(-96.9570275992017,-94.9970123582629,
177.685485069079));
#47114=CARTESIAN_POINT('Ctrl Pts',(-96.9570275996231,-94.9970123581598,
176.685485069079));
#47115=CARTESIAN_POINT('Ctrl Pts',(-95.5493747573727,-93.4257532338304,
177.685485069079));
#47116=CARTESIAN_POINT('Ctrl Pts',(-96.5209465833698,-93.1889913671421,
177.685485069079));
#47117=CARTESIAN_POINT('Ctrl Pts',(-96.5209465833055,-93.1889913671838,
176.685485069079));
#47118=CARTESIAN_POINT('Ctrl Pts',(-94.2152215208916,-88.0174687972257,
177.685485069079));
#47119=CARTESIAN_POINT('Ctrl Pts',(-95.18476174991,-87.7724714040589,177.685485069079));
#47120=CARTESIAN_POINT('Ctrl Pts',(-95.1847617500387,-87.7724714039756,
176.685485069079));
#47121=CARTESIAN_POINT('Ctrl Pts',(-93.2924266975675,-84.4230957726183,
177.685485069079));
#47122=CARTESIAN_POINT('Ctrl Pts',(-94.2595291227605,-84.1684584467021,
177.685485069079));
#47123=CARTESIAN_POINT('Ctrl Pts',(-94.259529122677,-84.1684584467251,176.685485069079));
#47124=CARTESIAN_POINT('Ctrl Pts',(-91.3239661578598,-77.2754177587244,
177.685485069079));
#47125=CARTESIAN_POINT('Ctrl Pts',(-92.2850778836019,-76.9990276012334,
177.685485069079));
#47126=CARTESIAN_POINT('Ctrl Pts',(-92.2850778836854,-76.9990276012104,
176.685485069079));
#47127=CARTESIAN_POINT('Ctrl Pts',(-90.2802592515923,-73.7220857400795,
177.685485069079));
#47128=CARTESIAN_POINT('Ctrl Pts',(-91.2377226352478,-73.433138928738,177.685485069079));
#47129=CARTESIAN_POINT('Ctrl Pts',(-91.2377226351847,-73.4331389287581,
176.685485069079));
#47130=CARTESIAN_POINT('Ctrl Pts',(-88.0433318090029,-66.6938040952403,
177.685485069079));
#47131=CARTESIAN_POINT('Ctrl Pts',(-88.9916685821912,-66.37618206286,177.685485069079));
#47132=CARTESIAN_POINT('Ctrl Pts',(-88.9916685822543,-66.3761820628399,
176.685485069079));
#47133=CARTESIAN_POINT('Ctrl Pts',(-86.849942999413,-63.2159635981179,177.685485069079));
#47134=CARTESIAN_POINT('Ctrl Pts',(-87.7928037540024,-62.8821750496115,
177.685485069079));
#47135=CARTESIAN_POINT('Ctrl Pts',(-87.7928037541667,-62.8821750495468,
176.685485069079));
#47136=CARTESIAN_POINT('Ctrl Pts',(-85.5577653075821,-59.7858708180287,
177.685485069079));
#47137=CARTESIAN_POINT('Ctrl Pts',(-86.4935648641577,-59.4333382806468,
177.685485069079));
#47138=CARTESIAN_POINT('Ctrl Pts',(-86.4935648641577,-59.4333382806468,
176.685485069079));
#47139=CARTESIAN_POINT('Origin',(-85.5577653075866,-59.7858708180409,176.685485069079));
#47140=CARTESIAN_POINT('Ctrl Pts',(-85.5194531411007,-59.8223115460841,
177.685438410949));
#47141=CARTESIAN_POINT('Ctrl Pts',(-86.4988068431487,-59.4471035664831,
177.735457988727));
#47142=CARTESIAN_POINT('Ctrl Pts',(-86.5441160166797,-59.5676907797451,
176.694509775823));
#47143=CARTESIAN_POINT('Ctrl Pts',(-85.5488285264639,-59.7938358236938,
177.685474105637));
#47144=CARTESIAN_POINT('Ctrl Pts',(-86.4967892966262,-59.4420366768795,
177.6973962827));
#47145=CARTESIAN_POINT('Ctrl Pts',(-86.499952014399,-59.4501665620726,176.678332308422));
#47146=CARTESIAN_POINT('Ctrl Pts',(-85.5871411152688,-59.7596096112386,
177.685523612831));
#47147=CARTESIAN_POINT('Ctrl Pts',(-86.4893362171423,-59.4220524652253,
177.646796562209));
#47148=CARTESIAN_POINT('Ctrl Pts',(-86.4548043581822,-59.3304223997585,
176.684724459335));
#47149=CARTESIAN_POINT('Ctrl Pts',(-85.6675280904232,-59.6585983136463,
177.68561487818));
#47150=CARTESIAN_POINT('Ctrl Pts',(-86.4551632269365,-59.3311831648032,
177.560550921871));
#47151=CARTESIAN_POINT('Ctrl Pts',(-86.3837085441107,-59.1424265153221,
176.72104467469));
#47152=CARTESIAN_POINT('Ctrl Pts',(-85.7032857420514,-59.609212897412,177.685652756804));
#47153=CARTESIAN_POINT('Ctrl Pts',(-86.4377267349023,-59.2848714957092,
177.527403265691));
#47154=CARTESIAN_POINT('Ctrl Pts',(-86.356803937052,-59.0714212354019,176.74128997663));
#47155=CARTESIAN_POINT('Ctrl Pts',(-85.7785946848509,-59.4648705863235,
177.685728562076));
#47156=CARTESIAN_POINT('Ctrl Pts',(-86.3883211207893,-59.1541829177556,
177.466627726095));
#47157=CARTESIAN_POINT('Ctrl Pts',(-86.3035833251825,-58.9312229886497,
176.788538683646));
#47158=CARTESIAN_POINT('Ctrl Pts',(-85.8199795319615,-59.369025485855,177.685766507573));
#47159=CARTESIAN_POINT('Ctrl Pts',(-86.3570787764338,-59.0717098514556,
177.439003405769));
#47160=CARTESIAN_POINT('Ctrl Pts',(-86.2773224730263,-58.8621727937877,
176.815857196747));
#47161=CARTESIAN_POINT('Ctrl Pts',(-85.8527453811609,-59.1638631347099,
177.685812659431));
#47162=CARTESIAN_POINT('Ctrl Pts',(-86.2952455717908,-58.9091065789535,
177.408732140999));
#47163=CARTESIAN_POINT('Ctrl Pts',(-86.237244648596,-58.7569891525569,176.851005000506));
#47164=CARTESIAN_POINT('Ctrl Pts',(-85.8580983310819,-59.0850699288534,
177.685825854228));
#47165=CARTESIAN_POINT('Ctrl Pts',(-86.2725674790216,-58.849546544774,177.400568011683));
#47166=CARTESIAN_POINT('Ctrl Pts',(-86.2237570173259,-58.7216236519169,
176.861619635495));
#47167=CARTESIAN_POINT('Ctrl Pts',(-85.8446620596993,-58.9106340093845,
177.685845148542));
#47168=CARTESIAN_POINT('Ctrl Pts',(-86.2230104183943,-58.7196046722724,
177.389314593047));
#47169=CARTESIAN_POINT('Ctrl Pts',(-86.1961425897331,-58.6492878843728,
176.87708230681));
#47170=CARTESIAN_POINT('Ctrl Pts',(-85.8247359731533,-58.8148969021221,
177.685850622447));
#47171=CARTESIAN_POINT('Ctrl Pts',(-86.1958236366334,-58.6484192889276,
177.386205525725));
#47172=CARTESIAN_POINT('Ctrl Pts',(-86.181985786926,-58.6122403466145,176.881690814559));
#47173=CARTESIAN_POINT('Ctrl Pts',(-85.757798456551,-58.6355045475111,177.685851182201));
#47174=CARTESIAN_POINT('Ctrl Pts',(-86.1425085870774,-58.5090309919607,
177.385885667039));
#47175=CARTESIAN_POINT('Ctrl Pts',(-86.1541477137945,-58.5394616866261,
176.882160986323));
#47176=CARTESIAN_POINT('Ctrl Pts',(-85.7111764310999,-58.5517673494884,
177.685846421581));
#47177=CARTESIAN_POINT('Ctrl Pts',(-86.1158285918039,-58.4393825623272,
177.388583808311));
#47178=CARTESIAN_POINT('Ctrl Pts',(-86.1403253895075,-58.5033607487595,
176.878144292243));
#47179=CARTESIAN_POINT('Ctrl Pts',(-85.6070035272959,-58.4105885808773,
177.685828410447));
#47180=CARTESIAN_POINT('Ctrl Pts',(-86.0659936678227,-58.3094686550687,
177.39904204685));
#47181=CARTESIAN_POINT('Ctrl Pts',(-86.1128226609236,-58.4315984586357,
176.86365543919));
#47182=CARTESIAN_POINT('Ctrl Pts',(-85.549953411443,-58.3529281116889,177.685815542119));
#47183=CARTESIAN_POINT('Ctrl Pts',(-86.0425829131345,-58.2485372045759,
177.406935364112));
#47184=CARTESIAN_POINT('Ctrl Pts',(-86.0991214598369,-58.3958830429589,
176.853266846028));
#47185=CARTESIAN_POINT('Ctrl Pts',(-85.3866542001269,-58.2165474304525,
177.685769931045));
#47186=CARTESIAN_POINT('Ctrl Pts',(-85.9787922610718,-58.0827294956763,
177.436623506163));
#47187=CARTESIAN_POINT('Ctrl Pts',(-86.0584515948782,-58.2899677801205,
176.818373491556));
#47188=CARTESIAN_POINT('Ctrl Pts',(-85.2896402982616,-58.1708177059058,
177.685731747951));
#47189=CARTESIAN_POINT('Ctrl Pts',(-85.9462013915549,-57.9983452958113,
177.46423345489));
#47190=CARTESIAN_POINT('Ctrl Pts',(-86.0316755766063,-58.220368101616,176.790702111615));
#47191=CARTESIAN_POINT('Ctrl Pts',(-85.1344296615373,-58.1114104723673,
177.685655451055));
#47192=CARTESIAN_POINT('Ctrl Pts',(-85.8946772447352,-57.8652228457512,
177.525111657089));
#47193=CARTESIAN_POINT('Ctrl Pts',(-85.9773869546852,-58.0795219938874,
176.74280243967));
#47194=CARTESIAN_POINT('Ctrl Pts',(-85.0738866036248,-58.0980831033533,
177.68561727497));
#47195=CARTESIAN_POINT('Ctrl Pts',(-85.8763844336074,-57.818157058371,177.558407398017));
#47196=CARTESIAN_POINT('Ctrl Pts',(-85.9499076944264,-58.0083634795133,
176.722185026019));
#47197=CARTESIAN_POINT('Ctrl Pts',(-84.9441455970151,-58.0757351762659,
177.685524740537));
#47198=CARTESIAN_POINT('Ctrl Pts',(-85.8402711553428,-57.7253572143701,
177.645672245051));
#47199=CARTESIAN_POINT('Ctrl Pts',(-85.8765913231287,-57.8188881891832,
176.684878031502));
#47200=CARTESIAN_POINT('Ctrl Pts',(-84.8918836039343,-58.0758297218312,
177.685474402246));
#47201=CARTESIAN_POINT('Ctrl Pts',(-85.8321927700424,-57.7047829333621,
177.697086633613));
#47202=CARTESIAN_POINT('Ctrl Pts',(-85.8297285808071,-57.6981502619506,
176.677860001849));
#47203=CARTESIAN_POINT('Ctrl Pts',(-84.8483096915888,-58.074185324701,177.685436168594));
#47204=CARTESIAN_POINT('Ctrl Pts',(-85.8301986118354,-57.6993383348146,
177.737896293016));
#47205=CARTESIAN_POINT('Ctrl Pts',(-85.7812152810651,-57.5735987346764,
176.695029611126));
#47206=CARTESIAN_POINT('Origin',(-84.9035795890714,-58.0758081979738,176.685485069078));
#47207=CARTESIAN_POINT('Ctrl Pts',(-84.9035795890714,-58.0758081979738,
177.685485069079));
#47208=CARTESIAN_POINT('Ctrl Pts',(-85.8357032382114,-57.7136680279926,
177.685485069079));
#47209=CARTESIAN_POINT('Ctrl Pts',(-85.8357032382114,-57.7136680279926,
176.685485069079));
#47210=CARTESIAN_POINT('Ctrl Pts',(-83.6957353880445,-54.9669011015685,
177.685485069079));
#47211=CARTESIAN_POINT('Ctrl Pts',(-84.6208766884138,-54.5867888507553,
177.685485069265));
#47212=CARTESIAN_POINT('Ctrl Pts',(-84.620876688336,-54.586788850792,176.685485069079));
#47213=CARTESIAN_POINT('Ctrl Pts',(-82.4022289102314,-51.899353553254,177.685485069079));
#47214=CARTESIAN_POINT('Ctrl Pts',(-83.3189771390602,-51.4990128922003,
177.685485069079));
#47215=CARTESIAN_POINT('Ctrl Pts',(-83.3189771388799,-51.4990128922617,
176.685485069079));
#47216=CARTESIAN_POINT('Ctrl Pts',(-80.2861211752646,-47.3832252372826,
177.685485069079));
#47217=CARTESIAN_POINT('Ctrl Pts',(-81.1860310864128,-46.9469487861368,
177.685485069079));
#47218=CARTESIAN_POINT('Ctrl Pts',(-81.1860310865029,-46.9469487861061,
176.685485069079));
#47219=CARTESIAN_POINT('Ctrl Pts',(-79.5512148812064,-45.8921459027875,
177.685485069079));
#47220=CARTESIAN_POINT('Ctrl Pts',(-80.4447931525142,-45.4429556181932,
177.68548506901));
#47221=CARTESIAN_POINT('Ctrl Pts',(-80.4447931524336,-45.4429556182301,
176.685485069033));
#47222=CARTESIAN_POINT('Ctrl Pts',(-78.3954041227117,-43.6813988570481,
177.685485069079));
#47223=CARTESIAN_POINT('Ctrl Pts',(-79.2779055104375,-43.2110215506448,
177.685485069114));
#47224=CARTESIAN_POINT('Ctrl Pts',(-79.2779055104779,-43.2110215506263,
176.685485069102));
#47225=CARTESIAN_POINT('Ctrl Pts',(-78.0011966023895,-42.9488090664747,
177.685485069079));
#47226=CARTESIAN_POINT('Ctrl Pts',(-78.8797401691368,-42.4710653373528,
177.685485069022));
#47227=CARTESIAN_POINT('Ctrl Pts',(-78.8797401690956,-42.4710653373763,
176.685485069033));
#47228=CARTESIAN_POINT('Ctrl Pts',(-77.3950072327152,-41.8571257984251,
177.685485069079));
#47229=CARTESIAN_POINT('Ctrl Pts',(-78.2671250050753,-41.3678098897351,
177.685485069108));
#47230=CARTESIAN_POINT('Ctrl Pts',(-78.267125005096,-41.3678098897234,176.685485069103));
#47231=CARTESIAN_POINT('Ctrl Pts',(-77.1904617586198,-41.4944329040509,
177.685485069079));
#47232=CARTESIAN_POINT('Ctrl Pts',(-78.0603558525197,-41.0011723956222,
177.685485069051));
#47233=CARTESIAN_POINT('Ctrl Pts',(-78.0603558525001,-41.0011723956339,
176.685485069056));
#47234=CARTESIAN_POINT('Ctrl Pts',(-76.776124475483,-40.7715864905627,177.685485069079));
#47235=CARTESIAN_POINT('Ctrl Pts',(-77.6413892786657,-40.270249793146,177.685485069108));
#47236=CARTESIAN_POINT('Ctrl Pts',(-77.6413892786852,-40.2702497931344,
176.685485069103));
#47237=CARTESIAN_POINT('Ctrl Pts',(-76.5654763654172,-40.4118964032511,
177.685485069079));
#47238=CARTESIAN_POINT('Ctrl Pts',(-77.427270789845,-39.904637716433,177.685485069079));
#47239=CARTESIAN_POINT('Ctrl Pts',(-77.4272707898366,-39.9046377164379,
176.685485069079));
#47240=CARTESIAN_POINT('Ctrl Pts',(-76.3543296174317,-40.0523497550927,
177.685485069079));
#47241=CARTESIAN_POINT('Ctrl Pts',(-77.2166317829811,-39.5459556642022,
177.685485069079));
#47242=CARTESIAN_POINT('Ctrl Pts',(-77.2166317829811,-39.5459556642022,
176.685485069079));
#47243=CARTESIAN_POINT('Ctrl Pts',(-85.5577653075812,-59.7858708180263,
174.285485069079));
#47244=CARTESIAN_POINT('Ctrl Pts',(-86.4935648641568,-59.4333382806444,
174.285485069079));
#47245=CARTESIAN_POINT('Ctrl Pts',(-86.4935648641568,-59.4333382806444,
175.285485069079));
#47246=CARTESIAN_POINT('Ctrl Pts',(-86.8499429992757,-63.2159635981751,
174.285485069079));
#47247=CARTESIAN_POINT('Ctrl Pts',(-87.7928037537602,-62.8821750497275,
174.285485068927));
#47248=CARTESIAN_POINT('Ctrl Pts',(-87.7928037541746,-62.8821750495676,
175.285485068927));
#47249=CARTESIAN_POINT('Ctrl Pts',(-88.0433318089691,-66.6938040952401,
174.285485069079));
#47250=CARTESIAN_POINT('Ctrl Pts',(-88.9916685821573,-66.3761820628341,
174.285485069079));
#47251=CARTESIAN_POINT('Ctrl Pts',(-88.9916685822437,-66.3761820628066,
175.285485069079));
#47252=CARTESIAN_POINT('Ctrl Pts',(-90.2802592516248,-73.7220857400759,
174.285485069079));
#47253=CARTESIAN_POINT('Ctrl Pts',(-91.2377226352804,-73.4331389287601,
174.285485069079));
#47254=CARTESIAN_POINT('Ctrl Pts',(-91.2377226351941,-73.4331389287876,
175.285485069079));
#47255=CARTESIAN_POINT('Ctrl Pts',(-91.3239661578861,-77.2754177587261,
174.285485069079));
#47256=CARTESIAN_POINT('Ctrl Pts',(-92.2850778836539,-76.9990276012609,
174.285485069079));
#47257=CARTESIAN_POINT('Ctrl Pts',(-92.2850778836961,-76.9990276012493,
175.285485069079));
#47258=CARTESIAN_POINT('Ctrl Pts',(-93.2924266975406,-84.423095772614,174.285485069079));
#47259=CARTESIAN_POINT('Ctrl Pts',(-94.2595291227079,-84.1684584466722,
174.285485069079));
#47260=CARTESIAN_POINT('Ctrl Pts',(-94.2595291226657,-84.1684584466838,
175.285485069079));
#47261=CARTESIAN_POINT('Ctrl Pts',(-94.2152215209114,-88.0174687973044,
174.285485069079));
#47262=CARTESIAN_POINT('Ctrl Pts',(-95.1847617499297,-87.772471404086,174.285485069079));
#47263=CARTESIAN_POINT('Ctrl Pts',(-95.1847617500581,-87.7724714040543,
175.285485069079));
#47264=CARTESIAN_POINT('Ctrl Pts',(-95.5493747573626,-93.4257532337901,
174.285485069079));
#47265=CARTESIAN_POINT('Ctrl Pts',(-96.5209465833597,-93.1889913671276,
174.285485069079));
#47266=CARTESIAN_POINT('Ctrl Pts',(-96.5209465832955,-93.1889913671434,
175.285485069079));
#47267=CARTESIAN_POINT('Ctrl Pts',(-95.9849221665606,-95.2315797810471,
174.285485069079));
#47268=CARTESIAN_POINT('Ctrl Pts',(-96.9570275991784,-94.997012358183,174.285485069079));
#47269=CARTESIAN_POINT('Ctrl Pts',(-96.9570275996033,-94.997012358079,175.285485069079));
#47270=CARTESIAN_POINT('Ctrl Pts',(-96.6472483679388,-97.9373097658926,
174.285485069079));
#47271=CARTESIAN_POINT('Ctrl Pts',(-97.618179127326,-97.6979435767939,174.285485069079));
#47272=CARTESIAN_POINT('Ctrl Pts',(-97.6181791271135,-97.6979435768459,
175.285485069079));
#47273=CARTESIAN_POINT('Ctrl Pts',(-96.8691183172565,-98.8388539217272,
174.285485069079));
#47274=CARTESIAN_POINT('Ctrl Pts',(-97.8394941595598,-98.5970607167033,
174.285485069079));
#47275=CARTESIAN_POINT('Ctrl Pts',(-97.8394941605458,-98.5970607164539,
175.285485069079));
#47276=CARTESIAN_POINT('Ctrl Pts',(-97.2185417746667,-100.185615621849,
174.285485069079));
#47277=CARTESIAN_POINT('Ctrl Pts',(-98.1852802927345,-99.9298032981384,
174.285485069079));
#47278=CARTESIAN_POINT('Ctrl Pts',(-98.1852802922415,-99.9298032982631,
175.285485069079));
#47279=CARTESIAN_POINT('Ctrl Pts',(-97.3376693870452,-100.633649414677,
174.285485069079));
#47280=CARTESIAN_POINT('Ctrl Pts',(-98.3028651239093,-100.371760565043,
174.285485069073));
#47281=CARTESIAN_POINT('Ctrl Pts',(-98.3028651257231,-100.371760564521,
175.285485069079));
#47282=CARTESIAN_POINT('Ctrl Pts',(-97.5287765043906,-101.301550314344,
174.285485069079));
#47283=CARTESIAN_POINT('Ctrl Pts',(-98.4883057294072,-101.019857554286,
174.285485069083));
#47284=CARTESIAN_POINT('Ctrl Pts',(-98.4883057285003,-101.019857554548,
175.285485069079));
#47285=CARTESIAN_POINT('Ctrl Pts',(-97.5945716173798,-101.523484475618,
174.285485069079));
#47286=CARTESIAN_POINT('Ctrl Pts',(-98.5516872373803,-101.233434821505,
174.285485069079));
#47287=CARTESIAN_POINT('Ctrl Pts',(-98.5516872395642,-101.23343482081,175.285485069079));
#47288=CARTESIAN_POINT('Ctrl Pts',(-97.6999002805479,-101.85416772093,174.285485069079));
#47289=CARTESIAN_POINT('Ctrl Pts',(-98.6505921303469,-101.543950403668,
174.285485069079));
#47290=CARTESIAN_POINT('Ctrl Pts',(-98.6505921292549,-101.543950404016,
175.285485069079));
#47291=CARTESIAN_POINT('Ctrl Pts',(-97.7361407722666,-101.964017467932,
174.285485069079));
#47292=CARTESIAN_POINT('Ctrl Pts',(-98.6842094799393,-101.645760425825,
174.285485069079));
#47293=CARTESIAN_POINT('Ctrl Pts',(-98.6842094816616,-101.645760425226,
175.285485069079));
#47294=CARTESIAN_POINT('Ctrl Pts',(-97.7931741603545,-102.127898788952,
174.285485069079));
#47295=CARTESIAN_POINT('Ctrl Pts',(-98.7358013339789,-101.794005894028,
174.285485069079));
#47296=CARTESIAN_POINT('Ctrl Pts',(-98.7358013331178,-101.794005894327,
175.285485069079));
#47297=CARTESIAN_POINT('Ctrl Pts',(-97.8126362132817,-102.182375180481,
174.285485069079));
#47298=CARTESIAN_POINT('Ctrl Pts',(-98.7531924801367,-101.842663688617,
174.285485069079));
#47299=CARTESIAN_POINT('Ctrl Pts',(-98.7531924811716,-101.842663688235,
175.285485069079));
#47300=CARTESIAN_POINT('Ctrl Pts',(-97.8527181088293,-102.290940987052,
174.285485069079));
#47301=CARTESIAN_POINT('Ctrl Pts',(-98.7883769389244,-101.937964302334,
174.285485069079));
#47302=CARTESIAN_POINT('Ctrl Pts',(-98.7883769378895,-101.937964302716,
175.285485069079));
#47303=CARTESIAN_POINT('Ctrl Pts',(-97.873036931237,-102.345134129228,174.285485069079));
#47304=CARTESIAN_POINT('Ctrl Pts',(-98.8109710951308,-101.998313235763,
174.285485069079));
#47305=CARTESIAN_POINT('Ctrl Pts',(-98.810971095131,-101.998313235765,175.285485069079));
#47306=CARTESIAN_POINT('Ctrl Pts',(-97.8932302579351,-102.399362986829,
174.285485069079));
#47307=CARTESIAN_POINT('Ctrl Pts',(-98.8303665270718,-102.050399359687,
174.285485069079));
#47308=CARTESIAN_POINT('Ctrl Pts',(-98.8303665270718,-102.050399359687,
175.285485069079));
#47309=CARTESIAN_POINT('Origin',(-85.5577653075812,-59.7858708180264,175.285485069079));
#47310=CARTESIAN_POINT('Ctrl Pts',(-86.549995003282,-59.5833376285491,175.274170498514));
#47311=CARTESIAN_POINT('Ctrl Pts',(-86.499087005688,-59.4478052525176,174.231213939548));
#47312=CARTESIAN_POINT('Ctrl Pts',(-85.5163014695733,-59.8258007915048,
174.285496900648));
#47313=CARTESIAN_POINT('Ctrl Pts',(-86.5039652636174,-59.4608115109789,
175.293174078778));
#47314=CARTESIAN_POINT('Ctrl Pts',(-86.4974436030401,-59.4437917418642,
174.269738655091));
#47315=CARTESIAN_POINT('Ctrl Pts',(-85.5461481361416,-59.7965609490947,
174.285488532754));
#47316=CARTESIAN_POINT('Ctrl Pts',(-86.4567528143649,-59.3355746263436,
175.287241072843));
#47317=CARTESIAN_POINT('Ctrl Pts',(-86.4902980810653,-59.4246102748182,
174.322388145275));
#47318=CARTESIAN_POINT('Ctrl Pts',(-85.5856213811138,-59.7621229158345,
174.28547663711));
#47319=CARTESIAN_POINT('Ctrl Pts',(-86.3837085441054,-59.1424265153082,
175.249925463467));
#47320=CARTESIAN_POINT('Ctrl Pts',(-86.4551137649122,-59.3310525045627,
174.411000335328));
#47321=CARTESIAN_POINT('Ctrl Pts',(-85.6681540564035,-59.6583380432654,
174.285454887567));
#47322=CARTESIAN_POINT('Ctrl Pts',(-86.356803937048,-59.0714212353912,175.229680161526));
#47323=CARTESIAN_POINT('Ctrl Pts',(-86.4376719251528,-59.2847269239036,
174.444099314138));
#47324=CARTESIAN_POINT('Ctrl Pts',(-85.703882282356,-59.6089493866821,174.285446138593));
#47325=CARTESIAN_POINT('Ctrl Pts',(-86.303583325178,-58.9312229886379,175.182431454508));
#47326=CARTESIAN_POINT('Ctrl Pts',(-86.3882664257975,-59.1540390056827,
174.504780092467));
#47327=CARTESIAN_POINT('Ctrl Pts',(-85.7791143736295,-59.4646057043272,
174.285428517499));
#47328=CARTESIAN_POINT('Ctrl Pts',(-86.2773224730233,-58.8621727937798,
175.155112941408));
#47329=CARTESIAN_POINT('Ctrl Pts',(-86.3570286560902,-59.0715781744698,
174.532358329031));
#47330=CARTESIAN_POINT('Ctrl Pts',(-85.8204497401368,-59.3687651284942,
174.285419843032));
#47331=CARTESIAN_POINT('Ctrl Pts',(-86.2372446485919,-58.756989152546,175.11996513765));
#47332=CARTESIAN_POINT('Ctrl Pts',(-86.2952103972096,-58.9090143275485,
174.562576229961));
#47333=CARTESIAN_POINT('Ctrl Pts',(-85.8531468169556,-59.1636319687109,
174.285409009404));
#47334=CARTESIAN_POINT('Ctrl Pts',(-86.2237570173223,-58.7216236519073,
175.109350502661));
#47335=CARTESIAN_POINT('Ctrl Pts',(-86.2725381980377,-58.849469804911,174.570725436989));
#47336=CARTESIAN_POINT('Ctrl Pts',(-85.8584784511242,-59.0848538815999,
174.285406058599));
#47337=CARTESIAN_POINT('Ctrl Pts',(-86.1961425897295,-58.6492878843634,
175.093887831347));
#47338=CARTESIAN_POINT('Ctrl Pts',(-86.2229945554986,-58.7195631569009,
174.581957969401));
#47339=CARTESIAN_POINT('Ctrl Pts',(-85.845014636378,-58.9104559691449,174.285401468371));
#47340=CARTESIAN_POINT('Ctrl Pts',(-86.1819857869222,-58.6122403466045,
175.089279323599));
#47341=CARTESIAN_POINT('Ctrl Pts',(-86.1958155063122,-58.6483980322719,
174.585061035853));
#47342=CARTESIAN_POINT('Ctrl Pts',(-85.8250834731818,-58.8147409947177,
174.285400256228));
#47343=CARTESIAN_POINT('Ctrl Pts',(-86.1541477137916,-58.5394616866186,
175.088809151837));
#47344=CARTESIAN_POINT('Ctrl Pts',(-86.142515422188,-58.5090488624724,174.585380285109));
#47345=CARTESIAN_POINT('Ctrl Pts',(-85.7581588973064,-58.6353860619252,
174.285400134323));
#47346=CARTESIAN_POINT('Ctrl Pts',(-86.1403253895043,-58.5033607487514,
175.092825845917));
#47347=CARTESIAN_POINT('Ctrl Pts',(-86.115843038762,-58.4394202933868,174.582687361069));
#47348=CARTESIAN_POINT('Ctrl Pts',(-85.7115539539042,-58.5516625188447,
174.285401185141));
#47349=CARTESIAN_POINT('Ctrl Pts',(-86.1128226609207,-58.431598458628,175.10731469897));
#47350=CARTESIAN_POINT('Ctrl Pts',(-86.0660217014019,-58.3095417665191,
174.572248593736));
#47351=CARTESIAN_POINT('Ctrl Pts',(-85.6074253887782,-58.4104956771806,
174.28540545462));
#47352=CARTESIAN_POINT('Ctrl Pts',(-86.0991214598344,-58.3958830429522,
175.117703292133));
#47353=CARTESIAN_POINT('Ctrl Pts',(-86.0426171221911,-58.2486263572438,
174.564369775238));
#47354=CARTESIAN_POINT('Ctrl Pts',(-85.5504013860293,-58.3528332272351,
174.28540834039));
#47355=CARTESIAN_POINT('Ctrl Pts',(-86.0584515948751,-58.2899677801124,
175.152596646605));
#47356=CARTESIAN_POINT('Ctrl Pts',(-85.9788421953099,-58.0828594024298,
174.534734180363));
#47357=CARTESIAN_POINT('Ctrl Pts',(-85.3871739388038,-58.2164300361061,
174.285419051878));
#47358=CARTESIAN_POINT('Ctrl Pts',(-86.0316755766042,-58.2203681016103,
175.180268026546));
#47359=CARTESIAN_POINT('Ctrl Pts',(-85.9462564441589,-57.9984882972759,
174.507170494432));
#47360=CARTESIAN_POINT('Ctrl Pts',(-85.2902011513818,-58.1706704423479,
174.285427777742));
#47361=CARTESIAN_POINT('Ctrl Pts',(-85.977386954683,-58.0795219938815,175.228167698491));
#47362=CARTESIAN_POINT('Ctrl Pts',(-85.8947331753262,-57.8653677607553,
174.446387500193));
#47363=CARTESIAN_POINT('Ctrl Pts',(-85.1350481968355,-58.11121024114,174.285445515549));
#47364=CARTESIAN_POINT('Ctrl Pts',(-85.949907694424,-58.0083634795072,175.248785112141));
#47365=CARTESIAN_POINT('Ctrl Pts',(-85.876435258962,-57.8182885447687,174.413140806164));
#47366=CARTESIAN_POINT('Ctrl Pts',(-85.0745252827981,-58.0978603796713,
174.285454331853));
#47367=CARTESIAN_POINT('Ctrl Pts',(-85.8745820102155,-57.8136954178983,
175.287114544409));
#47368=CARTESIAN_POINT('Ctrl Pts',(-85.8392537097024,-57.7227428207907,
174.32347969837));
#47369=CARTESIAN_POINT('Ctrl Pts',(-84.94126861619,-58.0748566531053,174.285476383955));
#47370=CARTESIAN_POINT('Ctrl Pts',(-85.8255622901349,-57.6874168715231,
175.29370201928));
#47371=CARTESIAN_POINT('Ctrl Pts',(-85.8314829454387,-57.702975857336,174.269971978808));
#47372=CARTESIAN_POINT('Ctrl Pts',(-84.8879909211494,-58.0755909926104,
174.285488480751));
#47373=CARTESIAN_POINT('Ctrl Pts',(-85.7747409433632,-57.5569792392174,
175.273508736808));
#47374=CARTESIAN_POINT('Ctrl Pts',(-85.8299220105362,-57.6985809329344,
174.228384991744));
#47375=CARTESIAN_POINT('Ctrl Pts',(-84.843264995634,-58.0736839758418,174.285497501802));
#47376=CARTESIAN_POINT('Origin',(-84.9035795890703,-58.0758081979709,175.285485069079));
#47377=CARTESIAN_POINT('Ctrl Pts',(-76.3543296174317,-40.0523497550927,
174.285485069079));
#47378=CARTESIAN_POINT('Ctrl Pts',(-77.2166317829811,-39.5459556642022,
174.285485069079));
#47379=CARTESIAN_POINT('Ctrl Pts',(-77.2166317829811,-39.5459556642022,
175.285485069079));
#47380=CARTESIAN_POINT('Ctrl Pts',(-76.5654763654227,-40.4118964032641,
174.285485069079));
#47381=CARTESIAN_POINT('Ctrl Pts',(-77.4272707898731,-39.9046377164337,
174.285485068964));
#47382=CARTESIAN_POINT('Ctrl Pts',(-77.4272707898438,-39.9046377164501,
175.285485068987));
#47383=CARTESIAN_POINT('Ctrl Pts',(-76.7761244754699,-40.7715864905485,
174.285485069079));
#47384=CARTESIAN_POINT('Ctrl Pts',(-77.6413892786381,-40.270249793139,174.285485069108));
#47385=CARTESIAN_POINT('Ctrl Pts',(-77.6413892786757,-40.2702497931179,
175.285485069103));
#47386=CARTESIAN_POINT('Ctrl Pts',(-77.1904617586327,-41.4944329040647,
174.285485069079));
#47387=CARTESIAN_POINT('Ctrl Pts',(-78.060355852547,-41.0011723956288,174.285485069051));
#47388=CARTESIAN_POINT('Ctrl Pts',(-78.0603558525094,-41.00117239565,175.285485069056));
#47389=CARTESIAN_POINT('Ctrl Pts',(-77.3950072327115,-41.8571257984251,
174.285485069079));
#47390=CARTESIAN_POINT('Ctrl Pts',(-78.2671250050659,-41.3678098897366,
174.285485069079));
#47391=CARTESIAN_POINT('Ctrl Pts',(-78.2671250050945,-41.3678098897207,
175.285485069079));
#47392=CARTESIAN_POINT('Ctrl Pts',(-78.0011966023962,-42.9488090664736,
174.285485069079));
#47393=CARTESIAN_POINT('Ctrl Pts',(-78.8797401691552,-42.4710653373489,
174.285485069079));
#47394=CARTESIAN_POINT('Ctrl Pts',(-78.879740169098,-42.4710653373806,175.285485069079));
#47395=CARTESIAN_POINT('Ctrl Pts',(-78.3954041226997,-43.68139885703,174.28548506908));
#47396=CARTESIAN_POINT('Ctrl Pts',(-79.277905510414,-43.2110215506354,174.28548506908));
#47397=CARTESIAN_POINT('Ctrl Pts',(-79.2779055104667,-43.2110215506049,
175.285485069079));
#47398=CARTESIAN_POINT('Ctrl Pts',(-79.5512148812292,-45.8921459028217,
174.28548506908));
#47399=CARTESIAN_POINT('Ctrl Pts',(-80.4447931525601,-45.4429556182101,
174.28548506908));
#47400=CARTESIAN_POINT('Ctrl Pts',(-80.4447931524548,-45.4429556182708,
175.285485069079));
#47401=CARTESIAN_POINT('Ctrl Pts',(-80.2861211753126,-47.3832252372925,
174.285485069079));
#47402=CARTESIAN_POINT('Ctrl Pts',(-81.1860310864378,-46.9469487861698,
174.285485069149));
#47403=CARTESIAN_POINT('Ctrl Pts',(-81.1860310865154,-46.9469487861327,
175.285485069126));
#47404=CARTESIAN_POINT('Ctrl Pts',(-82.4022289101332,-51.8993535532297,
174.285485069079));
#47405=CARTESIAN_POINT('Ctrl Pts',(-83.318977139008,-51.4990128921297,174.285485068941));
#47406=CARTESIAN_POINT('Ctrl Pts',(-83.3189771388528,-51.4990128922039,
175.285485068987));
#47407=CARTESIAN_POINT('Ctrl Pts',(-83.6957353882012,-54.9669011015501,
174.285485069079));
#47408=CARTESIAN_POINT('Ctrl Pts',(-84.6208766886056,-54.5867888507445,
174.285485068894));
#47409=CARTESIAN_POINT('Ctrl Pts',(-84.6208766883517,-54.5867888508327,
175.285485068894));
#47410=CARTESIAN_POINT('Ctrl Pts',(-84.9035795890702,-58.0758081979708,
174.285485069079));
#47411=CARTESIAN_POINT('Ctrl Pts',(-85.8357032382102,-57.7136680279897,
174.285485069079));
#47412=CARTESIAN_POINT('Ctrl Pts',(-85.8357032382102,-57.7136680279897,
175.285485069079));
#47701=UNCERTAINTY_MEASURE_WITH_UNIT(LENGTH_MEASURE(0.01),#47718,
'DISTANCE_ACCURACY_VALUE',
'Maximum model space distance between geometric entities at asserted c
onnectivities');
#47703=UNCERTAINTY_MEASURE_WITH_UNIT(LENGTH_MEASURE(0.01),#47718,
'DISTANCE_ACCURACY_VALUE',
'Maximum model space distance between geometric entities at asserted c
onnectivities');
#47715=(
GEOMETRIC_REPRESENTATION_CONTEXT(3)
GLOBAL_UNCERTAINTY_ASSIGNED_CONTEXT((#47701))
GLOBAL_UNIT_ASSIGNED_CONTEXT((#47718,#47720,#47721))
REPRESENTATION_CONTEXT('','3D')
);
#47717=(
GEOMETRIC_REPRESENTATION_CONTEXT(3)
GLOBAL_UNCERTAINTY_ASSIGNED_CONTEXT((#47703))
GLOBAL_UNIT_ASSIGNED_CONTEXT((#47718,#47720,#47721))
REPRESENTATION_CONTEXT('','3D')
);
#47718=(
LENGTH_UNIT()
NAMED_UNIT(*)
SI_UNIT(.MILLI.,.METRE.)
);
#47720=(
NAMED_UNIT(*)
PLANE_ANGLE_UNIT()
SI_UNIT($,.RADIAN.)
);
#47721=(
NAMED_UNIT(*)
SI_UNIT($,.STERADIAN.)
SOLID_ANGLE_UNIT()
);
#47733=SHAPE_DEFINITION_REPRESENTATION(#47746,#47771);
#47746=PRODUCT_DEFINITION_SHAPE('',$,#47785);
#47771=SHAPE_REPRESENTATION('',(#9834),#47715);
#47773=PRODUCT_DEFINITION_CONTEXT('part definition',#47814,'design');
#47785=PRODUCT_DEFINITION('Release Lever','Release Lever',#47798,#47773);
#47798=PRODUCT_DEFINITION_FORMATION('',$,#47827);
#47814=APPLICATION_CONTEXT(
'Core Data for Automotive Mechanical Design Process');
#47815=PRODUCT_CONTEXT('part definition',#47814,'mechanical');
#47827=PRODUCT('Release Lever','Release Lever',$,(#47815));
#47830=PRESENTATION_STYLE_ASSIGNMENT((#47832));
#47832=SURFACE_STYLE_USAGE(.BOTH.,#47834);
#47834=SURFACE_SIDE_STYLE('',(#47836));
#47836=SURFACE_STYLE_FILL_AREA(#47838);
#47838=FILL_AREA_STYLE('Opaque(202,209,238)',(#47840));
#47840=FILL_AREA_STYLE_COLOUR('Opaque(202,209,238)',#47842);
#47842=COLOUR_RGB('Opaque(202,209,238)', 0.66274510, 0.83137255, 0.94901961);
ENDSEC;
END-ISO-10303-21;
